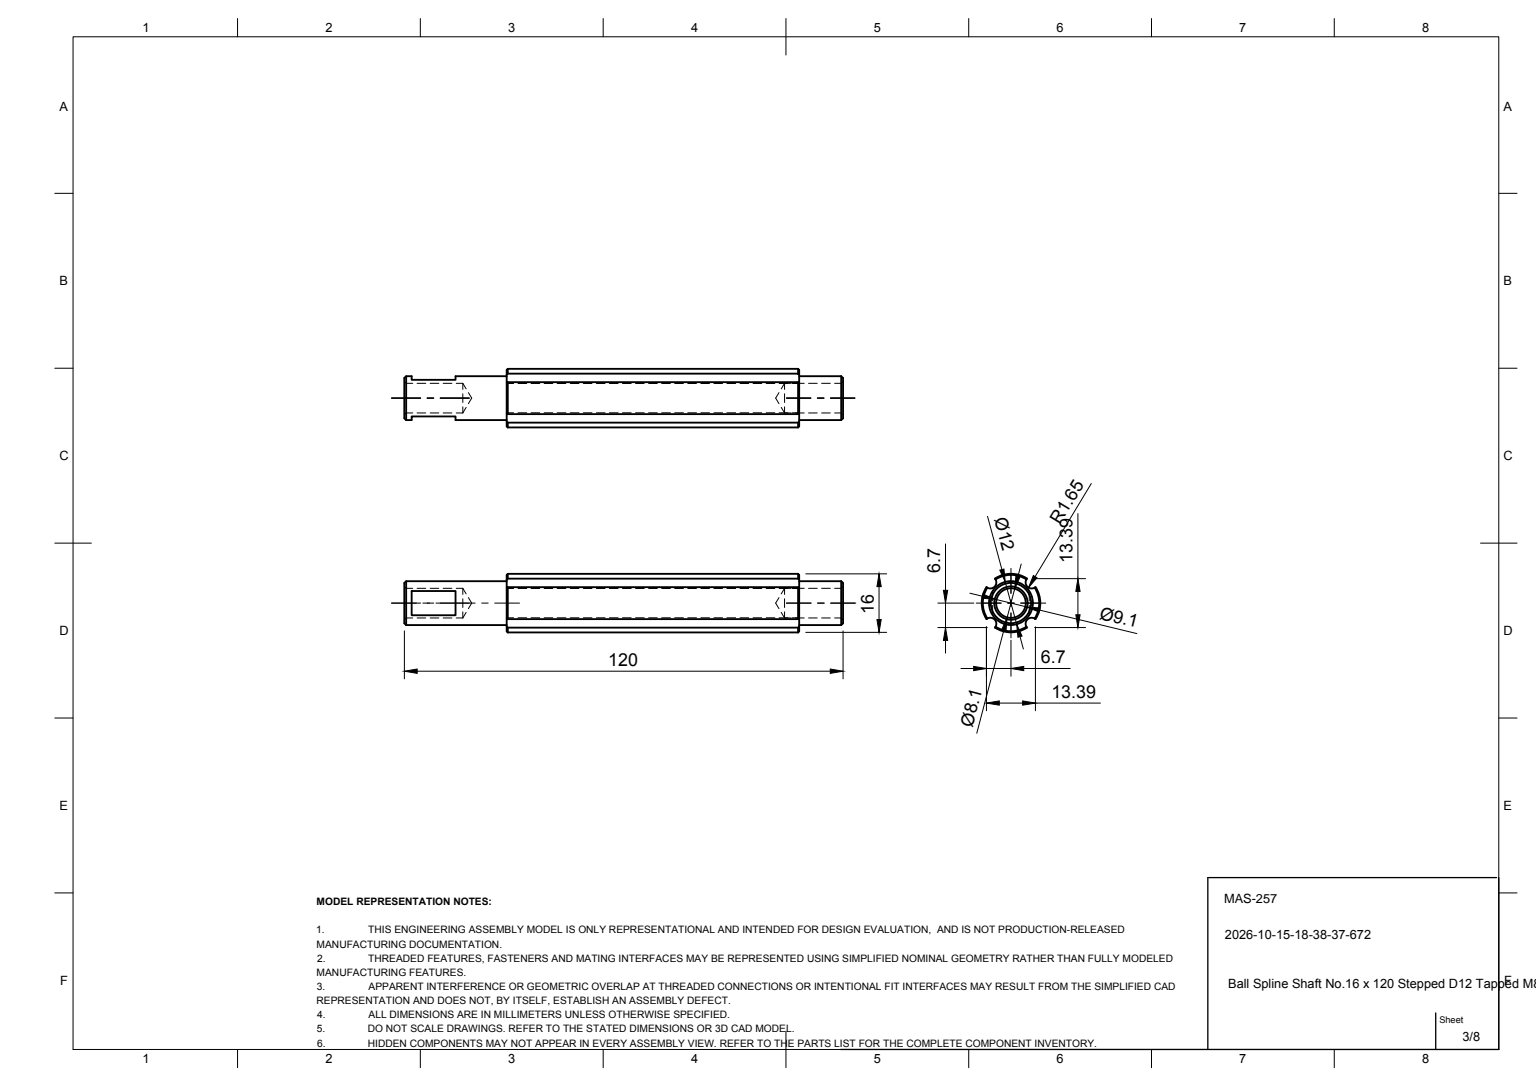
ISO-10303-21;
HEADER;
FILE_DESCRIPTION((''),'2;1');
FILE_NAME('Ball Spline Shaft No.16 x 120 Stepped D12 Tapped M8.step','2026-10-05T22:33:56+05:00',(''),(''),'','','');
FILE_SCHEMA (('AUTOMOTIVE_DESIGN { 1 0 10303 214 3 1 1 }'));
ENDSEC;
DATA;
#10=MECHANICAL_DESIGN_GEOMETRIC_PRESENTATION_REPRESENTATION('',(#429),#16942);
#415=SHAPE_REPRESENTATION_RELATIONSHIP('SRR','None',#17019,#422) ;
#422=ADVANCED_BREP_SHAPE_REPRESENTATION('',(#436),#16935) ;
#429=STYLED_ITEM('',(#17063),#436) ;
#436=MANIFOLD_SOLID_BREP(
'Ball Spline Shaft No.16 x 120 Stepped D12 Tapped M8',#8178) ;
#443=B_SPLINE_CURVE_WITH_KNOTS('',3,(#11023,#11024,#11025,#11026,#11027,
#11028),.UNSPECIFIED.,.F.,.F.,(4,2,4),(0.509460619201912,0.527252628402487,
0.551151897029291),.UNSPECIFIED.) ;
#444=B_SPLINE_CURVE_WITH_KNOTS('',3,(#11032,#11033,#11034,#11035,#11036,
#11037,#11038),.UNSPECIFIED.,.F.,.F.,(4,3,4),(-0.0238992690166207,0.,0.0177920092005774),
 .UNSPECIFIED.) ;
#445=B_SPLINE_CURVE_WITH_KNOTS('',3,(#11042,#11043,#11044,#11045,#11046,
#11047,#11048),.UNSPECIFIED.,.F.,.F.,(4,3,4),(-0.0177920090905049,0.,0.0238992686268042),
 .UNSPECIFIED.) ;
#446=B_SPLINE_CURVE_WITH_KNOTS('',3,(#11052,#11053,#11054,#11055,#11056,
#11057),.UNSPECIFIED.,.F.,.F.,(4,2,4),(0.660208716959523,0.684107985586327,
0.701899994786901),.UNSPECIFIED.) ;
#447=B_SPLINE_CURVE_WITH_KNOTS('',3,(#11062,#11063,#11064,#11065,#11066,
#11067),.UNSPECIFIED.,.F.,.F.,(4,2,4),(0.509460619201911,0.527252628402487,
0.55115189702929),.UNSPECIFIED.) ;
#448=B_SPLINE_CURVE_WITH_KNOTS('',3,(#11071,#11072,#11073,#11074,#11075,
#11076,#11077),.UNSPECIFIED.,.F.,.F.,(4,3,4),(-0.0238992690166204,0.,0.0177920092005756),
 .UNSPECIFIED.) ;
#449=B_SPLINE_CURVE_WITH_KNOTS('',3,(#11081,#11082,#11083,#11084,#11085,
#11086,#11087),.UNSPECIFIED.,.F.,.F.,(4,3,4),(-0.0177920090905051,0.,0.0238992686268041),
 .UNSPECIFIED.) ;
#450=B_SPLINE_CURVE_WITH_KNOTS('',3,(#11091,#11092,#11093,#11094,#11095,
#11096),.UNSPECIFIED.,.F.,.F.,(4,2,4),(0.660208716959522,0.684107985586326,
0.701899994786901),.UNSPECIFIED.) ;
#451=B_SPLINE_CURVE_WITH_KNOTS('',3,(#11101,#11102,#11103,#11104,#11105,
#11106,#11107),.UNSPECIFIED.,.F.,.F.,(4,3,4),(-0.0238992690166182,0.,0.0177920092005759),
 .UNSPECIFIED.) ;
#452=B_SPLINE_CURVE_WITH_KNOTS('',3,(#11111,#11112,#11113,#11114,#11115,
#11116,#11117),.UNSPECIFIED.,.F.,.F.,(4,3,4),(-0.0177920090905041,0.,0.0238992686268048),
 .UNSPECIFIED.) ;
#453=B_SPLINE_CURVE_WITH_KNOTS('',3,(#11121,#11122,#11123,#11124,#11125,
#11126),.UNSPECIFIED.,.F.,.F.,(4,2,4),(0.660208716959521,0.684107985586326,
0.701899994786899),.UNSPECIFIED.) ;
#454=B_SPLINE_CURVE_WITH_KNOTS('',3,(#11130,#11131,#11132,#11133,#11134,
#11135),.UNSPECIFIED.,.F.,.F.,(4,2,4),(0.509460619201914,0.52725262840249,
0.551151897029293),.UNSPECIFIED.) ;
#455=B_SPLINE_CURVE_WITH_KNOTS('',3,(#11140,#11141,#11142,#11143,#11144,
#11145,#11146),.UNSPECIFIED.,.F.,.F.,(4,3,4),(-0.0238992690166184,0.,0.0177920092005753),
 .UNSPECIFIED.) ;
#456=B_SPLINE_CURVE_WITH_KNOTS('',3,(#11150,#11151,#11152,#11153,#11154,
#11155,#11156),.UNSPECIFIED.,.F.,.F.,(4,3,4),(-0.0177920090905042,0.,0.0238992686268048),
 .UNSPECIFIED.) ;
#457=B_SPLINE_CURVE_WITH_KNOTS('',3,(#11160,#11161,#11162,#11163,#11164,
#11165),.UNSPECIFIED.,.F.,.F.,(4,2,4),(0.660208716959522,0.684107985586326,
0.7018999947869),.UNSPECIFIED.) ;
#458=B_SPLINE_CURVE_WITH_KNOTS('',3,(#11169,#11170,#11171,#11172,#11173,
#11174),.UNSPECIFIED.,.F.,.F.,(4,2,4),(0.509460619201915,0.527252628402489,
0.551151897029294),.UNSPECIFIED.) ;
#686=FACE_BOUND('',#1506,.T.) ;
#687=FACE_BOUND('',#1511,.T.) ;
#688=FACE_BOUND('',#1536,.T.) ;
#689=FACE_BOUND('',#1540,.T.) ;
#690=FACE_BOUND('',#1542,.T.) ;
#737=PLANE('',#8271) ;
#738=PLANE('',#8280) ;
#739=PLANE('',#8283) ;
#740=PLANE('',#8286) ;
#741=PLANE('',#8287) ;
#742=PLANE('',#8290) ;
#743=PLANE('',#8292) ;
#744=PLANE('',#8293) ;
#745=PLANE('',#8335) ;
#746=PLANE('',#8340) ;
#977=CYLINDRICAL_SURFACE('',#8268,4.05) ;
#978=CYLINDRICAL_SURFACE('',#8277,4.05) ;
#979=CYLINDRICAL_SURFACE('',#8295,1.65) ;
#980=CYLINDRICAL_SURFACE('',#8298,1.65) ;
#981=CYLINDRICAL_SURFACE('',#8301,1.65) ;
#982=CYLINDRICAL_SURFACE('',#8304,1.65) ;
#983=CYLINDRICAL_SURFACE('',#8319,8.) ;
#984=CYLINDRICAL_SURFACE('',#8321,8.) ;
#985=CYLINDRICAL_SURFACE('',#8323,8.) ;
#986=CYLINDRICAL_SURFACE('',#8325,8.) ;
#987=CYLINDRICAL_SURFACE('',#8339,6.) ;
#988=CYLINDRICAL_SURFACE('',#8342,6.) ;
#1061=FACE_OUTER_BOUND('',#1503,.T.) ;
#1062=FACE_OUTER_BOUND('',#1504,.T.) ;
#1063=FACE_OUTER_BOUND('',#1505,.T.) ;
#1064=FACE_OUTER_BOUND('',#1507,.T.) ;
#1065=FACE_OUTER_BOUND('',#1508,.T.) ;
#1066=FACE_OUTER_BOUND('',#1509,.T.) ;
#1067=FACE_OUTER_BOUND('',#1510,.T.) ;
#1068=FACE_OUTER_BOUND('',#1512,.T.) ;
#1069=FACE_OUTER_BOUND('',#1513,.T.) ;
#1070=FACE_OUTER_BOUND('',#1514,.T.) ;
#1071=FACE_OUTER_BOUND('',#1515,.T.) ;
#1072=FACE_OUTER_BOUND('',#1516,.T.) ;
#1073=FACE_OUTER_BOUND('',#1517,.T.) ;
#1074=FACE_OUTER_BOUND('',#1518,.T.) ;
#1075=FACE_OUTER_BOUND('',#1519,.T.) ;
#1076=FACE_OUTER_BOUND('',#1520,.T.) ;
#1077=FACE_OUTER_BOUND('',#1521,.T.) ;
#1078=FACE_OUTER_BOUND('',#1522,.T.) ;
#1079=FACE_OUTER_BOUND('',#1523,.T.) ;
#1080=FACE_OUTER_BOUND('',#1524,.T.) ;
#1081=FACE_OUTER_BOUND('',#1525,.T.) ;
#1082=FACE_OUTER_BOUND('',#1526,.T.) ;
#1083=FACE_OUTER_BOUND('',#1527,.T.) ;
#1084=FACE_OUTER_BOUND('',#1528,.T.) ;
#1085=FACE_OUTER_BOUND('',#1529,.T.) ;
#1086=FACE_OUTER_BOUND('',#1530,.T.) ;
#1087=FACE_OUTER_BOUND('',#1531,.T.) ;
#1088=FACE_OUTER_BOUND('',#1532,.T.) ;
#1089=FACE_OUTER_BOUND('',#1533,.T.) ;
#1090=FACE_OUTER_BOUND('',#1534,.T.) ;
#1091=FACE_OUTER_BOUND('',#1535,.T.) ;
#1092=FACE_OUTER_BOUND('',#1537,.T.) ;
#1093=FACE_OUTER_BOUND('',#1538,.T.) ;
#1094=FACE_OUTER_BOUND('',#1539,.T.) ;
#1095=FACE_OUTER_BOUND('',#1541,.T.) ;
#1096=FACE_OUTER_BOUND('',#1543,.T.) ;
#1503=EDGE_LOOP('',(#5351,#5352,#5353,#5354)) ;
#1504=EDGE_LOOP('',(#5355,#5356,#5357,#5358,#5359)) ;
#1505=EDGE_LOOP('',(#5360)) ;
#1506=EDGE_LOOP('',(#5361)) ;
#1507=EDGE_LOOP('',(#5362,#5363,#5364,#5365)) ;
#1508=EDGE_LOOP('',(#5366,#5367,#5368,#5369)) ;
#1509=EDGE_LOOP('',(#5370,#5371,#5372,#5373,#5374)) ;
#1510=EDGE_LOOP('',(#5375)) ;
#1511=EDGE_LOOP('',(#5376)) ;
#1512=EDGE_LOOP('',(#5377,#5378,#5379,#5380)) ;
#1513=EDGE_LOOP('',(#5381,#5382,#5383)) ;
#1514=EDGE_LOOP('',(#5384,#5385,#5386,#5387)) ;
#1515=EDGE_LOOP('',(#5388,#5389,#5390)) ;
#1516=EDGE_LOOP('',(#5391,#5392)) ;
#1517=EDGE_LOOP('',(#5393,#5394,#5395,#5396)) ;
#1518=EDGE_LOOP('',(#5397,#5398)) ;
#1519=EDGE_LOOP('',(#5399,#5400,#5401,#5402,#5403,#5404,#5405,#5406)) ;
#1520=EDGE_LOOP('',(#5407,#5408,#5409,#5410,#5411,#5412,#5413,#5414)) ;
#1521=EDGE_LOOP('',(#5415,#5416,#5417,#5418,#5419,#5420,#5421,#5422)) ;
#1522=EDGE_LOOP('',(#5423,#5424,#5425,#5426,#5427,#5428,#5429,#5430)) ;
#1523=EDGE_LOOP('',(#5431,#5432,#5433,#5434)) ;
#1524=EDGE_LOOP('',(#5435,#5436,#5437,#5438)) ;
#1525=EDGE_LOOP('',(#5439,#5440,#5441,#5442)) ;
#1526=EDGE_LOOP('',(#5443,#5444,#5445,#5446)) ;
#1527=EDGE_LOOP('',(#5447,#5448,#5449,#5450)) ;
#1528=EDGE_LOOP('',(#5451,#5452,#5453,#5454)) ;
#1529=EDGE_LOOP('',(#5455,#5456,#5457,#5458)) ;
#1530=EDGE_LOOP('',(#5459,#5460,#5461,#5462)) ;
#1531=EDGE_LOOP('',(#5463,#5464,#5465,#5466)) ;
#1532=EDGE_LOOP('',(#5467,#5468,#5469,#5470)) ;
#1533=EDGE_LOOP('',(#5471,#5472,#5473,#5474)) ;
#1534=EDGE_LOOP('',(#5475,#5476,#5477,#5478)) ;
#1535=EDGE_LOOP('',(#5479,#5480,#5481,#5482,#5483,#5484,#5485,#5486)) ;
#1536=EDGE_LOOP('',(#5487)) ;
#1537=EDGE_LOOP('',(#5488,#5489,#5490,#5491)) ;
#1538=EDGE_LOOP('',(#5492,#5493,#5494,#5495)) ;
#1539=EDGE_LOOP('',(#5496,#5497,#5498,#5499,#5500,#5501,#5502,#5503)) ;
#1540=EDGE_LOOP('',(#5504)) ;
#1541=EDGE_LOOP('',(#5505,#5506,#5507,#5508,#5509,#5510,#5511,#5512,#5513,
#5514,#5515,#5516)) ;
#1542=EDGE_LOOP('',(#5517,#5518,#5519,#5520)) ;
#1543=EDGE_LOOP('',(#5521,#5522,#5523,#5524)) ;
#1996=LINE('',#10958,#2558) ;
#1997=LINE('',#10962,#2559) ;
#1998=LINE('',#10971,#2560) ;
#1999=LINE('',#10976,#2561) ;
#2000=LINE('',#10980,#2562) ;
#2001=LINE('',#10989,#2563) ;
#2002=LINE('',#10995,#2564) ;
#2003=LINE('',#10999,#2565) ;
#2004=LINE('',#11001,#2566) ;
#2005=LINE('',#11002,#2567) ;
#2006=LINE('',#11011,#2568) ;
#2007=LINE('',#11014,#2569) ;
#2008=LINE('',#11016,#2570) ;
#2009=LINE('',#11017,#2571) ;
#2010=LINE('',#11040,#2572) ;
#2011=LINE('',#11058,#2573) ;
#2012=LINE('',#11079,#2574) ;
#2013=LINE('',#11097,#2575) ;
#2014=LINE('',#11109,#2576) ;
#2015=LINE('',#11128,#2577) ;
#2016=LINE('',#11148,#2578) ;
#2017=LINE('',#11167,#2579) ;
#2018=LINE('',#11210,#2580) ;
#2019=LINE('',#11212,#2581) ;
#2020=LINE('',#11219,#2582) ;
#2021=LINE('',#11220,#2583) ;
#2022=LINE('',#11222,#2584) ;
#2558=VECTOR('',#8980,4.3) ;
#2559=VECTOR('',#8985,4.05) ;
#2560=VECTOR('',#8996,2.025) ;
#2561=VECTOR('',#9001,4.3) ;
#2562=VECTOR('',#9006,4.05) ;
#2563=VECTOR('',#9017,4.05) ;
#2564=VECTOR('',#9022,10.) ;
#2565=VECTOR('',#9027,10.) ;
#2566=VECTOR('',#9028,10.) ;
#2567=VECTOR('',#9029,10.) ;
#2568=VECTOR('',#9040,10.) ;
#2569=VECTOR('',#9043,10.) ;
#2570=VECTOR('',#9044,10.) ;
#2571=VECTOR('',#9045,10.) ;
#2572=VECTOR('',#9054,10.) ;
#2573=VECTOR('',#9057,10.) ;
#2574=VECTOR('',#9062,10.) ;
#2575=VECTOR('',#9065,10.) ;
#2576=VECTOR('',#9068,10.) ;
#2577=VECTOR('',#9071,10.) ;
#2578=VECTOR('',#9076,10.) ;
#2579=VECTOR('',#9079,10.) ;
#2580=VECTOR('',#9146,5.75) ;
#2581=VECTOR('',#9149,6.) ;
#2582=VECTOR('',#9158,6.) ;
#2583=VECTOR('',#9159,6.) ;
#2584=VECTOR('',#9162,5.75) ;
#3120=CIRCLE('',#8266,4.55) ;
#3121=CIRCLE('',#8267,4.05) ;
#3122=CIRCLE('',#8269,4.05) ;
#3123=CIRCLE('',#8270,4.05) ;
#3124=CIRCLE('',#8272,5.5) ;
#3125=CIRCLE('',#8275,4.55) ;
#3126=CIRCLE('',#8276,4.05) ;
#3127=CIRCLE('',#8278,4.05) ;
#3128=CIRCLE('',#8279,4.05) ;
#3129=CIRCLE('',#8281,5.5) ;
#3130=CIRCLE('',#8284,6.) ;
#3131=CIRCLE('',#8285,6.) ;
#3132=CIRCLE('',#8288,6.) ;
#3133=CIRCLE('',#8289,6.) ;
#3134=CIRCLE('',#8291,6.) ;
#3135=CIRCLE('',#8294,6.) ;
#3136=CIRCLE('',#8296,1.65) ;
#3137=CIRCLE('',#8297,1.65) ;
#3138=CIRCLE('',#8299,1.65) ;
#3139=CIRCLE('',#8300,1.65) ;
#3140=CIRCLE('',#8302,1.65) ;
#3141=CIRCLE('',#8303,1.65) ;
#3142=CIRCLE('',#8305,1.65) ;
#3143=CIRCLE('',#8306,1.65) ;
#3144=CIRCLE('',#8308,8.) ;
#3145=CIRCLE('',#8309,7.7) ;
#3146=CIRCLE('',#8311,8.) ;
#3147=CIRCLE('',#8312,7.7) ;
#3148=CIRCLE('',#8314,7.7) ;
#3149=CIRCLE('',#8315,8.) ;
#3150=CIRCLE('',#8317,8.) ;
#3151=CIRCLE('',#8318,7.7) ;
#3152=CIRCLE('',#8320,8.) ;
#3153=CIRCLE('',#8322,8.) ;
#3154=CIRCLE('',#8324,8.) ;
#3155=CIRCLE('',#8326,8.) ;
#3156=CIRCLE('',#8328,7.7) ;
#3157=CIRCLE('',#8330,7.7) ;
#3158=CIRCLE('',#8332,7.7) ;
#3159=CIRCLE('',#8334,7.7) ;
#3160=CIRCLE('',#8336,6.) ;
#3161=CIRCLE('',#8338,6.) ;
#3162=CIRCLE('',#8341,6.) ;
#3163=CIRCLE('',#8343,6.) ;
#3398=VERTEX_POINT('',#10955) ;
#3399=VERTEX_POINT('',#10957) ;
#3400=VERTEX_POINT('',#10961) ;
#3401=VERTEX_POINT('',#10963) ;
#3402=VERTEX_POINT('',#10967) ;
#3403=VERTEX_POINT('',#10970) ;
#3404=VERTEX_POINT('',#10973) ;
#3405=VERTEX_POINT('',#10975) ;
#3406=VERTEX_POINT('',#10979) ;
#3407=VERTEX_POINT('',#10981) ;
#3408=VERTEX_POINT('',#10985) ;
#3409=VERTEX_POINT('',#10988) ;
#3410=VERTEX_POINT('',#10991) ;
#3411=VERTEX_POINT('',#10992) ;
#3412=VERTEX_POINT('',#10994) ;
#3413=VERTEX_POINT('',#10998) ;
#3414=VERTEX_POINT('',#11000) ;
#3415=VERTEX_POINT('',#11004) ;
#3416=VERTEX_POINT('',#11008) ;
#3417=VERTEX_POINT('',#11009) ;
#3418=VERTEX_POINT('',#11013) ;
#3419=VERTEX_POINT('',#11015) ;
#3420=VERTEX_POINT('',#11021) ;
#3421=VERTEX_POINT('',#11022) ;
#3422=VERTEX_POINT('',#11029) ;
#3423=VERTEX_POINT('',#11031) ;
#3424=VERTEX_POINT('',#11039) ;
#3425=VERTEX_POINT('',#11041) ;
#3426=VERTEX_POINT('',#11049) ;
#3427=VERTEX_POINT('',#11051) ;
#3428=VERTEX_POINT('',#11060) ;
#3429=VERTEX_POINT('',#11061) ;
#3430=VERTEX_POINT('',#11068) ;
#3431=VERTEX_POINT('',#11070) ;
#3432=VERTEX_POINT('',#11078) ;
#3433=VERTEX_POINT('',#11080) ;
#3434=VERTEX_POINT('',#11088) ;
#3435=VERTEX_POINT('',#11090) ;
#3436=VERTEX_POINT('',#11099) ;
#3437=VERTEX_POINT('',#11100) ;
#3438=VERTEX_POINT('',#11108) ;
#3439=VERTEX_POINT('',#11110) ;
#3440=VERTEX_POINT('',#11118) ;
#3441=VERTEX_POINT('',#11120) ;
#3442=VERTEX_POINT('',#11127) ;
#3443=VERTEX_POINT('',#11129) ;
#3444=VERTEX_POINT('',#11138) ;
#3445=VERTEX_POINT('',#11139) ;
#3446=VERTEX_POINT('',#11147) ;
#3447=VERTEX_POINT('',#11149) ;
#3448=VERTEX_POINT('',#11157) ;
#3449=VERTEX_POINT('',#11159) ;
#3450=VERTEX_POINT('',#11166) ;
#3451=VERTEX_POINT('',#11168) ;
#3452=VERTEX_POINT('',#11205) ;
#3453=VERTEX_POINT('',#11208) ;
#3454=VERTEX_POINT('',#11214) ;
#3455=VERTEX_POINT('',#11217) ;
#4173=EDGE_CURVE('',#3398,#3398,#3120,.T.) ;
#4174=EDGE_CURVE('',#3398,#3399,#1996,.T.) ;
#4175=EDGE_CURVE('',#3399,#3399,#3121,.T.) ;
#4176=EDGE_CURVE('',#3399,#3400,#1997,.T.) ;
#4177=EDGE_CURVE('',#3400,#3401,#3122,.T.) ;
#4178=EDGE_CURVE('',#3401,#3400,#3123,.T.) ;
#4179=EDGE_CURVE('',#3402,#3402,#3124,.T.) ;
#4180=EDGE_CURVE('',#3403,#3401,#1998,.T.) ;
#4181=EDGE_CURVE('',#3404,#3404,#3125,.T.) ;
#4182=EDGE_CURVE('',#3404,#3405,#1999,.T.) ;
#4183=EDGE_CURVE('',#3405,#3405,#3126,.T.) ;
#4184=EDGE_CURVE('',#3405,#3406,#2000,.T.) ;
#4185=EDGE_CURVE('',#3406,#3407,#3127,.T.) ;
#4186=EDGE_CURVE('',#3407,#3406,#3128,.T.) ;
#4187=EDGE_CURVE('',#3408,#3408,#3129,.T.) ;
#4188=EDGE_CURVE('',#3407,#3409,#2001,.T.) ;
#4189=EDGE_CURVE('',#3410,#3411,#3130,.T.) ;
#4190=EDGE_CURVE('',#3412,#3410,#2002,.T.) ;
#4191=EDGE_CURVE('',#3411,#3412,#3131,.T.) ;
#4192=EDGE_CURVE('',#3413,#3410,#2003,.T.) ;
#4193=EDGE_CURVE('',#3413,#3414,#2004,.T.) ;
#4194=EDGE_CURVE('',#3412,#3414,#2005,.T.) ;
#4195=EDGE_CURVE('',#3414,#3415,#3132,.T.) ;
#4196=EDGE_CURVE('',#3415,#3413,#3133,.T.) ;
#4197=EDGE_CURVE('',#3416,#3417,#3134,.T.) ;
#4198=EDGE_CURVE('',#3416,#3417,#2006,.T.) ;
#4199=EDGE_CURVE('',#3418,#3416,#2007,.T.) ;
#4200=EDGE_CURVE('',#3418,#3419,#2008,.T.) ;
#4201=EDGE_CURVE('',#3417,#3419,#2009,.T.) ;
#4202=EDGE_CURVE('',#3419,#3418,#3135,.T.) ;
#4203=EDGE_CURVE('',#3420,#3421,#443,.T.) ;
#4204=EDGE_CURVE('',#3422,#3420,#3136,.T.) ;
#4205=EDGE_CURVE('',#3423,#3422,#444,.T.) ;
#4206=EDGE_CURVE('',#3424,#3423,#2010,.T.) ;
#4207=EDGE_CURVE('',#3425,#3424,#445,.T.) ;
#4208=EDGE_CURVE('',#3426,#3425,#3137,.T.) ;
#4209=EDGE_CURVE('',#3427,#3426,#446,.T.) ;
#4210=EDGE_CURVE('',#3421,#3427,#2011,.T.) ;
#4211=EDGE_CURVE('',#3428,#3429,#447,.T.) ;
#4212=EDGE_CURVE('',#3430,#3428,#3138,.T.) ;
#4213=EDGE_CURVE('',#3431,#3430,#448,.T.) ;
#4214=EDGE_CURVE('',#3432,#3431,#2012,.T.) ;
#4215=EDGE_CURVE('',#3433,#3432,#449,.T.) ;
#4216=EDGE_CURVE('',#3434,#3433,#3139,.T.) ;
#4217=EDGE_CURVE('',#3435,#3434,#450,.T.) ;
#4218=EDGE_CURVE('',#3429,#3435,#2013,.T.) ;
#4219=EDGE_CURVE('',#3436,#3437,#451,.T.) ;
#4220=EDGE_CURVE('',#3438,#3436,#2014,.T.) ;
#4221=EDGE_CURVE('',#3439,#3438,#452,.T.) ;
#4222=EDGE_CURVE('',#3440,#3439,#3140,.T.) ;
#4223=EDGE_CURVE('',#3441,#3440,#453,.T.) ;
#4224=EDGE_CURVE('',#3442,#3441,#2015,.T.) ;
#4225=EDGE_CURVE('',#3443,#3442,#454,.T.) ;
#4226=EDGE_CURVE('',#3437,#3443,#3141,.T.) ;
#4227=EDGE_CURVE('',#3444,#3445,#455,.T.) ;
#4228=EDGE_CURVE('',#3446,#3444,#2016,.T.) ;
#4229=EDGE_CURVE('',#3447,#3446,#456,.T.) ;
#4230=EDGE_CURVE('',#3448,#3447,#3142,.T.) ;
#4231=EDGE_CURVE('',#3449,#3448,#457,.T.) ;
#4232=EDGE_CURVE('',#3450,#3449,#2017,.T.) ;
#4233=EDGE_CURVE('',#3451,#3450,#458,.T.) ;
#4234=EDGE_CURVE('',#3445,#3451,#3143,.T.) ;
#4235=EDGE_CURVE('',#3442,#3444,#3144,.T.) ;
#4236=EDGE_CURVE('',#3443,#3445,#3145,.T.) ;
#4237=EDGE_CURVE('',#3429,#3436,#3146,.T.) ;
#4238=EDGE_CURVE('',#3428,#3437,#3147,.T.) ;
#4239=EDGE_CURVE('',#3451,#3422,#3148,.T.) ;
#4240=EDGE_CURVE('',#3450,#3423,#3149,.T.) ;
#4241=EDGE_CURVE('',#3421,#3431,#3150,.T.) ;
#4242=EDGE_CURVE('',#3420,#3430,#3151,.T.) ;
#4243=EDGE_CURVE('',#3441,#3446,#3152,.T.) ;
#4244=EDGE_CURVE('',#3435,#3438,#3153,.T.) ;
#4245=EDGE_CURVE('',#3449,#3424,#3154,.T.) ;
#4246=EDGE_CURVE('',#3427,#3432,#3155,.T.) ;
#4247=EDGE_CURVE('',#3440,#3447,#3156,.T.) ;
#4248=EDGE_CURVE('',#3434,#3439,#3157,.T.) ;
#4249=EDGE_CURVE('',#3448,#3425,#3158,.T.) ;
#4250=EDGE_CURVE('',#3426,#3433,#3159,.T.) ;
#4251=EDGE_CURVE('',#3452,#3452,#3160,.T.) ;
#4252=EDGE_CURVE('',#3453,#3453,#3161,.T.) ;
#4253=EDGE_CURVE('',#3453,#3408,#2018,.T.) ;
#4254=EDGE_CURVE('',#3452,#3453,#2019,.T.) ;
#4255=EDGE_CURVE('',#3454,#3454,#3162,.T.) ;
#4256=EDGE_CURVE('',#3455,#3455,#3163,.T.) ;
#4257=EDGE_CURVE('',#3455,#3411,#2020,.T.) ;
#4258=EDGE_CURVE('',#3415,#3454,#2021,.T.) ;
#4259=EDGE_CURVE('',#3402,#3455,#2022,.T.) ;
#5351=ORIENTED_EDGE('',*,*,#4173,.T.) ;
#5352=ORIENTED_EDGE('',*,*,#4174,.T.) ;
#5353=ORIENTED_EDGE('',*,*,#4175,.T.) ;
#5354=ORIENTED_EDGE('',*,*,#4174,.F.) ;
#5355=ORIENTED_EDGE('',*,*,#4175,.F.) ;
#5356=ORIENTED_EDGE('',*,*,#4176,.T.) ;
#5357=ORIENTED_EDGE('',*,*,#4177,.T.) ;
#5358=ORIENTED_EDGE('',*,*,#4178,.T.) ;
#5359=ORIENTED_EDGE('',*,*,#4176,.F.) ;
#5360=ORIENTED_EDGE('',*,*,#4179,.T.) ;
#5361=ORIENTED_EDGE('',*,*,#4173,.F.) ;
#5362=ORIENTED_EDGE('',*,*,#4180,.T.) ;
#5363=ORIENTED_EDGE('',*,*,#4177,.F.) ;
#5364=ORIENTED_EDGE('',*,*,#4178,.F.) ;
#5365=ORIENTED_EDGE('',*,*,#4180,.F.) ;
#5366=ORIENTED_EDGE('',*,*,#4181,.T.) ;
#5367=ORIENTED_EDGE('',*,*,#4182,.T.) ;
#5368=ORIENTED_EDGE('',*,*,#4183,.T.) ;
#5369=ORIENTED_EDGE('',*,*,#4182,.F.) ;
#5370=ORIENTED_EDGE('',*,*,#4183,.F.) ;
#5371=ORIENTED_EDGE('',*,*,#4184,.T.) ;
#5372=ORIENTED_EDGE('',*,*,#4185,.T.) ;
#5373=ORIENTED_EDGE('',*,*,#4186,.T.) ;
#5374=ORIENTED_EDGE('',*,*,#4184,.F.) ;
#5375=ORIENTED_EDGE('',*,*,#4187,.F.) ;
#5376=ORIENTED_EDGE('',*,*,#4181,.F.) ;
#5377=ORIENTED_EDGE('',*,*,#4186,.F.) ;
#5378=ORIENTED_EDGE('',*,*,#4188,.T.) ;
#5379=ORIENTED_EDGE('',*,*,#4188,.F.) ;
#5380=ORIENTED_EDGE('',*,*,#4185,.F.) ;
#5381=ORIENTED_EDGE('',*,*,#4189,.F.) ;
#5382=ORIENTED_EDGE('',*,*,#4190,.F.) ;
#5383=ORIENTED_EDGE('',*,*,#4191,.F.) ;
#5384=ORIENTED_EDGE('',*,*,#4192,.F.) ;
#5385=ORIENTED_EDGE('',*,*,#4193,.T.) ;
#5386=ORIENTED_EDGE('',*,*,#4194,.F.) ;
#5387=ORIENTED_EDGE('',*,*,#4190,.T.) ;
#5388=ORIENTED_EDGE('',*,*,#4195,.F.) ;
#5389=ORIENTED_EDGE('',*,*,#4193,.F.) ;
#5390=ORIENTED_EDGE('',*,*,#4196,.F.) ;
#5391=ORIENTED_EDGE('',*,*,#4197,.F.) ;
#5392=ORIENTED_EDGE('',*,*,#4198,.T.) ;
#5393=ORIENTED_EDGE('',*,*,#4199,.F.) ;
#5394=ORIENTED_EDGE('',*,*,#4200,.T.) ;
#5395=ORIENTED_EDGE('',*,*,#4201,.F.) ;
#5396=ORIENTED_EDGE('',*,*,#4198,.F.) ;
#5397=ORIENTED_EDGE('',*,*,#4202,.F.) ;
#5398=ORIENTED_EDGE('',*,*,#4200,.F.) ;
#5399=ORIENTED_EDGE('',*,*,#4203,.F.) ;
#5400=ORIENTED_EDGE('',*,*,#4204,.F.) ;
#5401=ORIENTED_EDGE('',*,*,#4205,.F.) ;
#5402=ORIENTED_EDGE('',*,*,#4206,.F.) ;
#5403=ORIENTED_EDGE('',*,*,#4207,.F.) ;
#5404=ORIENTED_EDGE('',*,*,#4208,.F.) ;
#5405=ORIENTED_EDGE('',*,*,#4209,.F.) ;
#5406=ORIENTED_EDGE('',*,*,#4210,.F.) ;
#5407=ORIENTED_EDGE('',*,*,#4211,.F.) ;
#5408=ORIENTED_EDGE('',*,*,#4212,.F.) ;
#5409=ORIENTED_EDGE('',*,*,#4213,.F.) ;
#5410=ORIENTED_EDGE('',*,*,#4214,.F.) ;
#5411=ORIENTED_EDGE('',*,*,#4215,.F.) ;
#5412=ORIENTED_EDGE('',*,*,#4216,.F.) ;
#5413=ORIENTED_EDGE('',*,*,#4217,.F.) ;
#5414=ORIENTED_EDGE('',*,*,#4218,.F.) ;
#5415=ORIENTED_EDGE('',*,*,#4219,.F.) ;
#5416=ORIENTED_EDGE('',*,*,#4220,.F.) ;
#5417=ORIENTED_EDGE('',*,*,#4221,.F.) ;
#5418=ORIENTED_EDGE('',*,*,#4222,.F.) ;
#5419=ORIENTED_EDGE('',*,*,#4223,.F.) ;
#5420=ORIENTED_EDGE('',*,*,#4224,.F.) ;
#5421=ORIENTED_EDGE('',*,*,#4225,.F.) ;
#5422=ORIENTED_EDGE('',*,*,#4226,.F.) ;
#5423=ORIENTED_EDGE('',*,*,#4227,.F.) ;
#5424=ORIENTED_EDGE('',*,*,#4228,.F.) ;
#5425=ORIENTED_EDGE('',*,*,#4229,.F.) ;
#5426=ORIENTED_EDGE('',*,*,#4230,.F.) ;
#5427=ORIENTED_EDGE('',*,*,#4231,.F.) ;
#5428=ORIENTED_EDGE('',*,*,#4232,.F.) ;
#5429=ORIENTED_EDGE('',*,*,#4233,.F.) ;
#5430=ORIENTED_EDGE('',*,*,#4234,.F.) ;
#5431=ORIENTED_EDGE('',*,*,#4225,.T.) ;
#5432=ORIENTED_EDGE('',*,*,#4235,.T.) ;
#5433=ORIENTED_EDGE('',*,*,#4227,.T.) ;
#5434=ORIENTED_EDGE('',*,*,#4236,.F.) ;
#5435=ORIENTED_EDGE('',*,*,#4211,.T.) ;
#5436=ORIENTED_EDGE('',*,*,#4237,.T.) ;
#5437=ORIENTED_EDGE('',*,*,#4219,.T.) ;
#5438=ORIENTED_EDGE('',*,*,#4238,.F.) ;
#5439=ORIENTED_EDGE('',*,*,#4205,.T.) ;
#5440=ORIENTED_EDGE('',*,*,#4239,.F.) ;
#5441=ORIENTED_EDGE('',*,*,#4233,.T.) ;
#5442=ORIENTED_EDGE('',*,*,#4240,.T.) ;
#5443=ORIENTED_EDGE('',*,*,#4203,.T.) ;
#5444=ORIENTED_EDGE('',*,*,#4241,.T.) ;
#5445=ORIENTED_EDGE('',*,*,#4213,.T.) ;
#5446=ORIENTED_EDGE('',*,*,#4242,.F.) ;
#5447=ORIENTED_EDGE('',*,*,#4224,.T.) ;
#5448=ORIENTED_EDGE('',*,*,#4243,.T.) ;
#5449=ORIENTED_EDGE('',*,*,#4228,.T.) ;
#5450=ORIENTED_EDGE('',*,*,#4235,.F.) ;
#5451=ORIENTED_EDGE('',*,*,#4218,.T.) ;
#5452=ORIENTED_EDGE('',*,*,#4244,.T.) ;
#5453=ORIENTED_EDGE('',*,*,#4220,.T.) ;
#5454=ORIENTED_EDGE('',*,*,#4237,.F.) ;
#5455=ORIENTED_EDGE('',*,*,#4206,.T.) ;
#5456=ORIENTED_EDGE('',*,*,#4240,.F.) ;
#5457=ORIENTED_EDGE('',*,*,#4232,.T.) ;
#5458=ORIENTED_EDGE('',*,*,#4245,.T.) ;
#5459=ORIENTED_EDGE('',*,*,#4210,.T.) ;
#5460=ORIENTED_EDGE('',*,*,#4246,.T.) ;
#5461=ORIENTED_EDGE('',*,*,#4214,.T.) ;
#5462=ORIENTED_EDGE('',*,*,#4241,.F.) ;
#5463=ORIENTED_EDGE('',*,*,#4223,.T.) ;
#5464=ORIENTED_EDGE('',*,*,#4247,.T.) ;
#5465=ORIENTED_EDGE('',*,*,#4229,.T.) ;
#5466=ORIENTED_EDGE('',*,*,#4243,.F.) ;
#5467=ORIENTED_EDGE('',*,*,#4217,.T.) ;
#5468=ORIENTED_EDGE('',*,*,#4248,.T.) ;
#5469=ORIENTED_EDGE('',*,*,#4221,.T.) ;
#5470=ORIENTED_EDGE('',*,*,#4244,.F.) ;
#5471=ORIENTED_EDGE('',*,*,#4207,.T.) ;
#5472=ORIENTED_EDGE('',*,*,#4245,.F.) ;
#5473=ORIENTED_EDGE('',*,*,#4231,.T.) ;
#5474=ORIENTED_EDGE('',*,*,#4249,.T.) ;
#5475=ORIENTED_EDGE('',*,*,#4209,.T.) ;
#5476=ORIENTED_EDGE('',*,*,#4250,.T.) ;
#5477=ORIENTED_EDGE('',*,*,#4215,.T.) ;
#5478=ORIENTED_EDGE('',*,*,#4246,.F.) ;
#5479=ORIENTED_EDGE('',*,*,#4208,.T.) ;
#5480=ORIENTED_EDGE('',*,*,#4249,.F.) ;
#5481=ORIENTED_EDGE('',*,*,#4230,.T.) ;
#5482=ORIENTED_EDGE('',*,*,#4247,.F.) ;
#5483=ORIENTED_EDGE('',*,*,#4222,.T.) ;
#5484=ORIENTED_EDGE('',*,*,#4248,.F.) ;
#5485=ORIENTED_EDGE('',*,*,#4216,.T.) ;
#5486=ORIENTED_EDGE('',*,*,#4250,.F.) ;
#5487=ORIENTED_EDGE('',*,*,#4251,.T.) ;
#5488=ORIENTED_EDGE('',*,*,#4252,.F.) ;
#5489=ORIENTED_EDGE('',*,*,#4253,.T.) ;
#5490=ORIENTED_EDGE('',*,*,#4187,.T.) ;
#5491=ORIENTED_EDGE('',*,*,#4253,.F.) ;
#5492=ORIENTED_EDGE('',*,*,#4251,.F.) ;
#5493=ORIENTED_EDGE('',*,*,#4254,.T.) ;
#5494=ORIENTED_EDGE('',*,*,#4252,.T.) ;
#5495=ORIENTED_EDGE('',*,*,#4254,.F.) ;
#5496=ORIENTED_EDGE('',*,*,#4204,.T.) ;
#5497=ORIENTED_EDGE('',*,*,#4242,.T.) ;
#5498=ORIENTED_EDGE('',*,*,#4212,.T.) ;
#5499=ORIENTED_EDGE('',*,*,#4238,.T.) ;
#5500=ORIENTED_EDGE('',*,*,#4226,.T.) ;
#5501=ORIENTED_EDGE('',*,*,#4236,.T.) ;
#5502=ORIENTED_EDGE('',*,*,#4234,.T.) ;
#5503=ORIENTED_EDGE('',*,*,#4239,.T.) ;
#5504=ORIENTED_EDGE('',*,*,#4255,.F.) ;
#5505=ORIENTED_EDGE('',*,*,#4256,.F.) ;
#5506=ORIENTED_EDGE('',*,*,#4257,.T.) ;
#5507=ORIENTED_EDGE('',*,*,#4191,.T.) ;
#5508=ORIENTED_EDGE('',*,*,#4194,.T.) ;
#5509=ORIENTED_EDGE('',*,*,#4195,.T.) ;
#5510=ORIENTED_EDGE('',*,*,#4258,.T.) ;
#5511=ORIENTED_EDGE('',*,*,#4255,.T.) ;
#5512=ORIENTED_EDGE('',*,*,#4258,.F.) ;
#5513=ORIENTED_EDGE('',*,*,#4196,.T.) ;
#5514=ORIENTED_EDGE('',*,*,#4192,.T.) ;
#5515=ORIENTED_EDGE('',*,*,#4189,.T.) ;
#5516=ORIENTED_EDGE('',*,*,#4257,.F.) ;
#5517=ORIENTED_EDGE('',*,*,#4201,.T.) ;
#5518=ORIENTED_EDGE('',*,*,#4202,.T.) ;
#5519=ORIENTED_EDGE('',*,*,#4199,.T.) ;
#5520=ORIENTED_EDGE('',*,*,#4197,.T.) ;
#5521=ORIENTED_EDGE('',*,*,#4179,.F.) ;
#5522=ORIENTED_EDGE('',*,*,#4259,.T.) ;
#5523=ORIENTED_EDGE('',*,*,#4256,.T.) ;
#5524=ORIENTED_EDGE('',*,*,#4259,.F.) ;
#7707=CONICAL_SURFACE('',#8265,4.3,0.785398163397439) ;
#7708=CONICAL_SURFACE('',#8273,2.025,1.02974425867665) ;
#7709=CONICAL_SURFACE('',#8274,4.3,0.785398163397447) ;
#7710=CONICAL_SURFACE('',#8282,4.05,1.02974425867666) ;
#7711=CONICAL_SURFACE('',#8307,7.85,0.785398163397456) ;
#7712=CONICAL_SURFACE('',#8310,7.85,0.785398163397456) ;
#7713=CONICAL_SURFACE('',#8313,7.85,0.785398163397456) ;
#7714=CONICAL_SURFACE('',#8316,7.85,0.785398163397456) ;
#7715=CONICAL_SURFACE('',#8327,7.85,0.785398163397445) ;
#7716=CONICAL_SURFACE('',#8329,7.85,0.785398163397445) ;
#7717=CONICAL_SURFACE('',#8331,7.85,0.785398163397445) ;
#7718=CONICAL_SURFACE('',#8333,7.85,0.785398163397445) ;
#7719=CONICAL_SURFACE('',#8337,5.75,0.785398163397447) ;
#7720=CONICAL_SURFACE('',#8344,5.75,0.785398163397439) ;
#7736=ADVANCED_FACE('',(#1061),#7707,.F.) ;
#7737=ADVANCED_FACE('',(#1062),#977,.F.) ;
#7738=ADVANCED_FACE('',(#1063,#686),#737,.T.) ;
#7739=ADVANCED_FACE('',(#1064),#7708,.F.) ;
#7740=ADVANCED_FACE('',(#1065),#7709,.F.) ;
#7741=ADVANCED_FACE('',(#1066),#978,.F.) ;
#7742=ADVANCED_FACE('',(#1067,#687),#738,.T.) ;
#7743=ADVANCED_FACE('',(#1068),#7710,.F.) ;
#7744=ADVANCED_FACE('',(#1069),#739,.F.) ;
#7745=ADVANCED_FACE('',(#1070),#740,.F.) ;
#7746=ADVANCED_FACE('',(#1071),#741,.T.) ;
#7747=ADVANCED_FACE('',(#1072),#742,.T.) ;
#7748=ADVANCED_FACE('',(#1073),#743,.F.) ;
#7749=ADVANCED_FACE('',(#1074),#744,.F.) ;
#7750=ADVANCED_FACE('',(#1075),#979,.F.) ;
#7751=ADVANCED_FACE('',(#1076),#980,.F.) ;
#7752=ADVANCED_FACE('',(#1077),#981,.F.) ;
#7753=ADVANCED_FACE('',(#1078),#982,.F.) ;
#7754=ADVANCED_FACE('',(#1079),#7711,.T.) ;
#7755=ADVANCED_FACE('',(#1080),#7712,.T.) ;
#7756=ADVANCED_FACE('',(#1081),#7713,.T.) ;
#7757=ADVANCED_FACE('',(#1082),#7714,.T.) ;
#7758=ADVANCED_FACE('',(#1083),#983,.T.) ;
#7759=ADVANCED_FACE('',(#1084),#984,.T.) ;
#7760=ADVANCED_FACE('',(#1085),#985,.T.) ;
#7761=ADVANCED_FACE('',(#1086),#986,.T.) ;
#7762=ADVANCED_FACE('',(#1087),#7715,.T.) ;
#7763=ADVANCED_FACE('',(#1088),#7716,.T.) ;
#7764=ADVANCED_FACE('',(#1089),#7717,.T.) ;
#7765=ADVANCED_FACE('',(#1090),#7718,.T.) ;
#7766=ADVANCED_FACE('',(#1091,#688),#745,.T.) ;
#7767=ADVANCED_FACE('',(#1092),#7719,.T.) ;
#7768=ADVANCED_FACE('',(#1093),#987,.T.) ;
#7769=ADVANCED_FACE('',(#1094,#689),#746,.T.) ;
#7770=ADVANCED_FACE('',(#1095,#690),#988,.T.) ;
#7771=ADVANCED_FACE('',(#1096),#7720,.T.) ;
#8178=CLOSED_SHELL('',(#7736,#7737,#7738,#7739,#7740,#7741,#7742,#7743,
#7744,#7745,#7746,#7747,#7748,#7749,#7750,#7751,#7752,#7753,#7754,#7755,
#7756,#7757,#7758,#7759,#7760,#7761,#7762,#7763,#7764,#7765,#7766,#7767,
#7768,#7769,#7770,#7771)) ;
#8264=AXIS2_PLACEMENT_3D('',#10953,#8974,#8975) ;
#8265=AXIS2_PLACEMENT_3D('',#10954,#8976,#8977) ;
#8266=AXIS2_PLACEMENT_3D('',#10956,#8978,#8979) ;
#8267=AXIS2_PLACEMENT_3D('',#10959,#8981,#8982) ;
#8268=AXIS2_PLACEMENT_3D('',#10960,#8983,#8984) ;
#8269=AXIS2_PLACEMENT_3D('',#10964,#8986,#8987) ;
#8270=AXIS2_PLACEMENT_3D('',#10965,#8988,#8989) ;
#8271=AXIS2_PLACEMENT_3D('',#10966,#8990,#8991) ;
#8272=AXIS2_PLACEMENT_3D('',#10968,#8992,#8993) ;
#8273=AXIS2_PLACEMENT_3D('',#10969,#8994,#8995) ;
#8274=AXIS2_PLACEMENT_3D('',#10972,#8997,#8998) ;
#8275=AXIS2_PLACEMENT_3D('',#10974,#8999,#9000) ;
#8276=AXIS2_PLACEMENT_3D('',#10977,#9002,#9003) ;
#8277=AXIS2_PLACEMENT_3D('',#10978,#9004,#9005) ;
#8278=AXIS2_PLACEMENT_3D('',#10982,#9007,#9008) ;
#8279=AXIS2_PLACEMENT_3D('',#10983,#9009,#9010) ;
#8280=AXIS2_PLACEMENT_3D('',#10984,#9011,#9012) ;
#8281=AXIS2_PLACEMENT_3D('',#10986,#9013,#9014) ;
#8282=AXIS2_PLACEMENT_3D('',#10987,#9015,#9016) ;
#8283=AXIS2_PLACEMENT_3D('',#10990,#9018,#9019) ;
#8284=AXIS2_PLACEMENT_3D('',#10993,#9020,#9021) ;
#8285=AXIS2_PLACEMENT_3D('',#10996,#9023,#9024) ;
#8286=AXIS2_PLACEMENT_3D('',#10997,#9025,#9026) ;
#8287=AXIS2_PLACEMENT_3D('',#11003,#9030,#9031) ;
#8288=AXIS2_PLACEMENT_3D('',#11005,#9032,#9033) ;
#8289=AXIS2_PLACEMENT_3D('',#11006,#9034,#9035) ;
#8290=AXIS2_PLACEMENT_3D('',#11007,#9036,#9037) ;
#8291=AXIS2_PLACEMENT_3D('',#11010,#9038,#9039) ;
#8292=AXIS2_PLACEMENT_3D('',#11012,#9041,#9042) ;
#8293=AXIS2_PLACEMENT_3D('',#11018,#9046,#9047) ;
#8294=AXIS2_PLACEMENT_3D('',#11019,#9048,#9049) ;
#8295=AXIS2_PLACEMENT_3D('',#11020,#9050,#9051) ;
#8296=AXIS2_PLACEMENT_3D('',#11030,#9052,#9053) ;
#8297=AXIS2_PLACEMENT_3D('',#11050,#9055,#9056) ;
#8298=AXIS2_PLACEMENT_3D('',#11059,#9058,#9059) ;
#8299=AXIS2_PLACEMENT_3D('',#11069,#9060,#9061) ;
#8300=AXIS2_PLACEMENT_3D('',#11089,#9063,#9064) ;
#8301=AXIS2_PLACEMENT_3D('',#11098,#9066,#9067) ;
#8302=AXIS2_PLACEMENT_3D('',#11119,#9069,#9070) ;
#8303=AXIS2_PLACEMENT_3D('',#11136,#9072,#9073) ;
#8304=AXIS2_PLACEMENT_3D('',#11137,#9074,#9075) ;
#8305=AXIS2_PLACEMENT_3D('',#11158,#9077,#9078) ;
#8306=AXIS2_PLACEMENT_3D('',#11175,#9080,#9081) ;
#8307=AXIS2_PLACEMENT_3D('',#11176,#9082,#9083) ;
#8308=AXIS2_PLACEMENT_3D('',#11177,#9084,#9085) ;
#8309=AXIS2_PLACEMENT_3D('',#11178,#9086,#9087) ;
#8310=AXIS2_PLACEMENT_3D('',#11179,#9088,#9089) ;
#8311=AXIS2_PLACEMENT_3D('',#11180,#9090,#9091) ;
#8312=AXIS2_PLACEMENT_3D('',#11181,#9092,#9093) ;
#8313=AXIS2_PLACEMENT_3D('',#11182,#9094,#9095) ;
#8314=AXIS2_PLACEMENT_3D('',#11183,#9096,#9097) ;
#8315=AXIS2_PLACEMENT_3D('',#11184,#9098,#9099) ;
#8316=AXIS2_PLACEMENT_3D('',#11185,#9100,#9101) ;
#8317=AXIS2_PLACEMENT_3D('',#11186,#9102,#9103) ;
#8318=AXIS2_PLACEMENT_3D('',#11187,#9104,#9105) ;
#8319=AXIS2_PLACEMENT_3D('',#11188,#9106,#9107) ;
#8320=AXIS2_PLACEMENT_3D('',#11189,#9108,#9109) ;
#8321=AXIS2_PLACEMENT_3D('',#11190,#9110,#9111) ;
#8322=AXIS2_PLACEMENT_3D('',#11191,#9112,#9113) ;
#8323=AXIS2_PLACEMENT_3D('',#11192,#9114,#9115) ;
#8324=AXIS2_PLACEMENT_3D('',#11193,#9116,#9117) ;
#8325=AXIS2_PLACEMENT_3D('',#11194,#9118,#9119) ;
#8326=AXIS2_PLACEMENT_3D('',#11195,#9120,#9121) ;
#8327=AXIS2_PLACEMENT_3D('',#11196,#9122,#9123) ;
#8328=AXIS2_PLACEMENT_3D('',#11197,#9124,#9125) ;
#8329=AXIS2_PLACEMENT_3D('',#11198,#9126,#9127) ;
#8330=AXIS2_PLACEMENT_3D('',#11199,#9128,#9129) ;
#8331=AXIS2_PLACEMENT_3D('',#11200,#9130,#9131) ;
#8332=AXIS2_PLACEMENT_3D('',#11201,#9132,#9133) ;
#8333=AXIS2_PLACEMENT_3D('',#11202,#9134,#9135) ;
#8334=AXIS2_PLACEMENT_3D('',#11203,#9136,#9137) ;
#8335=AXIS2_PLACEMENT_3D('',#11204,#9138,#9139) ;
#8336=AXIS2_PLACEMENT_3D('',#11206,#9140,#9141) ;
#8337=AXIS2_PLACEMENT_3D('',#11207,#9142,#9143) ;
#8338=AXIS2_PLACEMENT_3D('',#11209,#9144,#9145) ;
#8339=AXIS2_PLACEMENT_3D('',#11211,#9147,#9148) ;
#8340=AXIS2_PLACEMENT_3D('',#11213,#9150,#9151) ;
#8341=AXIS2_PLACEMENT_3D('',#11215,#9152,#9153) ;
#8342=AXIS2_PLACEMENT_3D('',#11216,#9154,#9155) ;
#8343=AXIS2_PLACEMENT_3D('',#11218,#9156,#9157) ;
#8344=AXIS2_PLACEMENT_3D('',#11221,#9160,#9161) ;
#8974=DIRECTION('axis',(0.,0.,1.)) ;
#8975=DIRECTION('refdir',(1.,0.,0.)) ;
#8976=DIRECTION('center_axis',(1.,0.,0.)) ;
#8977=DIRECTION('ref_axis',(0.,0.,-1.)) ;
#8978=DIRECTION('center_axis',(1.,0.,0.)) ;
#8979=DIRECTION('ref_axis',(0.,0.,-1.)) ;
#8980=DIRECTION('',(-0.707106781186554,8.65956056235486E-17,-0.707106781186541)) ;
#8981=DIRECTION('center_axis',(-1.,0.,0.)) ;
#8982=DIRECTION('ref_axis',(0.,0.,-1.)) ;
#8983=DIRECTION('center_axis',(-1.,0.,0.)) ;
#8984=DIRECTION('ref_axis',(0.,0.,-1.)) ;
#8985=DIRECTION('',(-1.,0.,0.)) ;
#8986=DIRECTION('center_axis',(-1.,0.,0.)) ;
#8987=DIRECTION('ref_axis',(0.,0.,-1.)) ;
#8988=DIRECTION('center_axis',(-1.,0.,0.)) ;
#8989=DIRECTION('ref_axis',(0.,0.,-1.)) ;
#8990=DIRECTION('center_axis',(1.,0.,0.)) ;
#8991=DIRECTION('ref_axis',(0.,0.,-1.)) ;
#8992=DIRECTION('center_axis',(1.,0.,0.)) ;
#8993=DIRECTION('ref_axis',(0.,0.,-1.)) ;
#8994=DIRECTION('center_axis',(1.,0.,0.)) ;
#8995=DIRECTION('ref_axis',(0.,1.,0.)) ;
#8996=DIRECTION('',(0.515038074910055,-0.857167300702112,-1.04972719113862E-16)) ;
#8997=DIRECTION('center_axis',(-1.,0.,0.)) ;
#8998=DIRECTION('ref_axis',(0.,0.,-1.)) ;
#8999=DIRECTION('center_axis',(-1.,0.,0.)) ;
#9000=DIRECTION('ref_axis',(0.,0.,-1.)) ;
#9001=DIRECTION('',(0.707106781186549,-8.65956056235492E-17,-0.707106781186546)) ;
#9002=DIRECTION('center_axis',(1.,0.,0.)) ;
#9003=DIRECTION('ref_axis',(0.,0.,-1.)) ;
#9004=DIRECTION('center_axis',(1.,0.,0.)) ;
#9005=DIRECTION('ref_axis',(0.,0.,-1.)) ;
#9006=DIRECTION('',(1.,0.,0.)) ;
#9007=DIRECTION('center_axis',(1.,0.,0.)) ;
#9008=DIRECTION('ref_axis',(0.,0.,-1.)) ;
#9009=DIRECTION('center_axis',(1.,0.,0.)) ;
#9010=DIRECTION('ref_axis',(0.,0.,-1.)) ;
#9011=DIRECTION('center_axis',(-1.,0.,0.)) ;
#9012=DIRECTION('ref_axis',(0.,0.,1.)) ;
#9013=DIRECTION('center_axis',(1.,0.,0.)) ;
#9014=DIRECTION('ref_axis',(0.,0.,-1.)) ;
#9015=DIRECTION('center_axis',(-1.,0.,0.)) ;
#9016=DIRECTION('ref_axis',(0.,1.,0.)) ;
#9017=DIRECTION('',(0.515038074910053,0.857167300702113,1.04972719113862E-16)) ;
#9018=DIRECTION('center_axis',(1.,0.,0.)) ;
#9019=DIRECTION('ref_axis',(0.,0.,-1.)) ;
#9020=DIRECTION('center_axis',(1.,0.,0.)) ;
#9021=DIRECTION('ref_axis',(0.,1.,0.)) ;
#9022=DIRECTION('',(0.,0.,1.)) ;
#9023=DIRECTION('center_axis',(1.,0.,0.)) ;
#9024=DIRECTION('ref_axis',(0.,1.,0.)) ;
#9025=DIRECTION('center_axis',(0.,1.,0.)) ;
#9026=DIRECTION('ref_axis',(0.,0.,1.)) ;
#9027=DIRECTION('',(1.,0.,0.)) ;
#9028=DIRECTION('',(0.,0.,-1.)) ;
#9029=DIRECTION('',(-1.,0.,0.)) ;
#9030=DIRECTION('center_axis',(1.,0.,0.)) ;
#9031=DIRECTION('ref_axis',(0.,0.,-1.)) ;
#9032=DIRECTION('center_axis',(-1.,0.,0.)) ;
#9033=DIRECTION('ref_axis',(0.,1.,0.)) ;
#9034=DIRECTION('center_axis',(-1.,0.,0.)) ;
#9035=DIRECTION('ref_axis',(0.,1.,0.)) ;
#9036=DIRECTION('center_axis',(1.,0.,0.)) ;
#9037=DIRECTION('ref_axis',(0.,0.,-1.)) ;
#9038=DIRECTION('center_axis',(-1.,0.,0.)) ;
#9039=DIRECTION('ref_axis',(0.,1.,0.)) ;
#9040=DIRECTION('',(0.,0.,-1.)) ;
#9041=DIRECTION('center_axis',(0.,-1.,0.)) ;
#9042=DIRECTION('ref_axis',(0.,0.,-1.)) ;
#9043=DIRECTION('',(-1.,0.,0.)) ;
#9044=DIRECTION('',(0.,0.,-1.)) ;
#9045=DIRECTION('',(1.,0.,0.)) ;
#9046=DIRECTION('center_axis',(1.,0.,0.)) ;
#9047=DIRECTION('ref_axis',(0.,0.,-1.)) ;
#9048=DIRECTION('center_axis',(1.,0.,0.)) ;
#9049=DIRECTION('ref_axis',(0.,1.,0.)) ;
#9050=DIRECTION('center_axis',(1.,0.,0.)) ;
#9051=DIRECTION('ref_axis',(0.,0.707106781186547,0.707106781186548)) ;
#9052=DIRECTION('center_axis',(-1.,0.,0.)) ;
#9053=DIRECTION('ref_axis',(0.,0.,-1.)) ;
#9054=DIRECTION('',(1.,0.,0.)) ;
#9055=DIRECTION('center_axis',(1.,0.,0.)) ;
#9056=DIRECTION('ref_axis',(0.,0.,-1.)) ;
#9057=DIRECTION('',(-1.,0.,0.)) ;
#9058=DIRECTION('center_axis',(1.,0.,0.)) ;
#9059=DIRECTION('ref_axis',(0.,-0.707106781186547,0.707106781186548)) ;
#9060=DIRECTION('center_axis',(-1.,0.,0.)) ;
#9061=DIRECTION('ref_axis',(0.,0.,-1.)) ;
#9062=DIRECTION('',(1.,0.,0.)) ;
#9063=DIRECTION('center_axis',(1.,0.,0.)) ;
#9064=DIRECTION('ref_axis',(0.,0.,-1.)) ;
#9065=DIRECTION('',(-1.,0.,0.)) ;
#9066=DIRECTION('center_axis',(1.,0.,0.)) ;
#9067=DIRECTION('ref_axis',(0.,0.,-1.)) ;
#9068=DIRECTION('',(1.,0.,0.)) ;
#9069=DIRECTION('center_axis',(1.,0.,0.)) ;
#9070=DIRECTION('ref_axis',(0.,0.,-1.)) ;
#9071=DIRECTION('',(-1.,0.,0.)) ;
#9072=DIRECTION('center_axis',(-1.,0.,0.)) ;
#9073=DIRECTION('ref_axis',(0.,0.,-1.)) ;
#9074=DIRECTION('center_axis',(1.,0.,0.)) ;
#9075=DIRECTION('ref_axis',(0.,0.,-1.)) ;
#9076=DIRECTION('',(1.,0.,0.)) ;
#9077=DIRECTION('center_axis',(1.,0.,0.)) ;
#9078=DIRECTION('ref_axis',(0.,0.,-1.)) ;
#9079=DIRECTION('',(-1.,0.,0.)) ;
#9080=DIRECTION('center_axis',(-1.,0.,0.)) ;
#9081=DIRECTION('ref_axis',(0.,0.,-1.)) ;
#9082=DIRECTION('center_axis',(-1.,0.,0.)) ;
#9083=DIRECTION('ref_axis',(0.,1.,0.)) ;
#9084=DIRECTION('center_axis',(1.,0.,0.)) ;
#9085=DIRECTION('ref_axis',(0.,0.,-1.)) ;
#9086=DIRECTION('center_axis',(1.,0.,0.)) ;
#9087=DIRECTION('ref_axis',(0.,0.,-1.)) ;
#9088=DIRECTION('center_axis',(-1.,0.,0.)) ;
#9089=DIRECTION('ref_axis',(0.,1.,0.)) ;
#9090=DIRECTION('center_axis',(1.,0.,0.)) ;
#9091=DIRECTION('ref_axis',(0.,0.,-1.)) ;
#9092=DIRECTION('center_axis',(1.,0.,0.)) ;
#9093=DIRECTION('ref_axis',(0.,0.,-1.)) ;
#9094=DIRECTION('center_axis',(-1.,0.,0.)) ;
#9095=DIRECTION('ref_axis',(0.,-1.,-1.01064309961486E-15)) ;
#9096=DIRECTION('center_axis',(1.,0.,0.)) ;
#9097=DIRECTION('ref_axis',(0.,0.,-1.)) ;
#9098=DIRECTION('center_axis',(1.,0.,0.)) ;
#9099=DIRECTION('ref_axis',(0.,0.,-1.)) ;
#9100=DIRECTION('center_axis',(-1.,0.,0.)) ;
#9101=DIRECTION('ref_axis',(0.,1.,0.)) ;
#9102=DIRECTION('center_axis',(1.,0.,0.)) ;
#9103=DIRECTION('ref_axis',(0.,0.,-1.)) ;
#9104=DIRECTION('center_axis',(1.,0.,0.)) ;
#9105=DIRECTION('ref_axis',(0.,0.,-1.)) ;
#9106=DIRECTION('center_axis',(1.,0.,0.)) ;
#9107=DIRECTION('ref_axis',(0.,1.,0.)) ;
#9108=DIRECTION('center_axis',(1.,0.,0.)) ;
#9109=DIRECTION('ref_axis',(0.,0.,-1.)) ;
#9110=DIRECTION('center_axis',(1.,0.,0.)) ;
#9111=DIRECTION('ref_axis',(0.,1.,0.)) ;
#9112=DIRECTION('center_axis',(1.,0.,0.)) ;
#9113=DIRECTION('ref_axis',(0.,0.,-1.)) ;
#9114=DIRECTION('center_axis',(1.,0.,0.)) ;
#9115=DIRECTION('ref_axis',(0.,-1.,-1.01064309961486E-15)) ;
#9116=DIRECTION('center_axis',(1.,0.,0.)) ;
#9117=DIRECTION('ref_axis',(0.,0.,-1.)) ;
#9118=DIRECTION('center_axis',(1.,0.,0.)) ;
#9119=DIRECTION('ref_axis',(0.,1.,0.)) ;
#9120=DIRECTION('center_axis',(1.,0.,0.)) ;
#9121=DIRECTION('ref_axis',(0.,0.,-1.)) ;
#9122=DIRECTION('center_axis',(1.,0.,0.)) ;
#9123=DIRECTION('ref_axis',(0.,1.,0.)) ;
#9124=DIRECTION('center_axis',(1.,0.,0.)) ;
#9125=DIRECTION('ref_axis',(0.,0.,-1.)) ;
#9126=DIRECTION('center_axis',(1.,0.,0.)) ;
#9127=DIRECTION('ref_axis',(0.,1.,0.)) ;
#9128=DIRECTION('center_axis',(1.,0.,0.)) ;
#9129=DIRECTION('ref_axis',(0.,0.,-1.)) ;
#9130=DIRECTION('center_axis',(1.,0.,0.)) ;
#9131=DIRECTION('ref_axis',(0.,-1.,-1.01064309961486E-15)) ;
#9132=DIRECTION('center_axis',(1.,0.,0.)) ;
#9133=DIRECTION('ref_axis',(0.,0.,-1.)) ;
#9134=DIRECTION('center_axis',(1.,0.,0.)) ;
#9135=DIRECTION('ref_axis',(0.,1.,0.)) ;
#9136=DIRECTION('center_axis',(1.,0.,0.)) ;
#9137=DIRECTION('ref_axis',(0.,0.,-1.)) ;
#9138=DIRECTION('center_axis',(-1.,0.,0.)) ;
#9139=DIRECTION('ref_axis',(0.,0.,1.)) ;
#9140=DIRECTION('center_axis',(1.,0.,0.)) ;
#9141=DIRECTION('ref_axis',(0.,0.,-1.)) ;
#9142=DIRECTION('center_axis',(1.,0.,0.)) ;
#9143=DIRECTION('ref_axis',(0.,1.,0.)) ;
#9144=DIRECTION('center_axis',(1.,0.,0.)) ;
#9145=DIRECTION('ref_axis',(0.,0.,-1.)) ;
#9146=DIRECTION('',(-0.707106781186549,0.707106781186546,8.65956056235492E-17)) ;
#9147=DIRECTION('center_axis',(1.,0.,0.)) ;
#9148=DIRECTION('ref_axis',(0.,1.,0.)) ;
#9149=DIRECTION('',(-1.,0.,0.)) ;
#9150=DIRECTION('center_axis',(1.,0.,0.)) ;
#9151=DIRECTION('ref_axis',(0.,0.,-1.)) ;
#9152=DIRECTION('center_axis',(1.,0.,0.)) ;
#9153=DIRECTION('ref_axis',(0.,0.,-1.)) ;
#9154=DIRECTION('center_axis',(1.,0.,0.)) ;
#9155=DIRECTION('ref_axis',(0.,1.,0.)) ;
#9156=DIRECTION('center_axis',(1.,0.,0.)) ;
#9157=DIRECTION('ref_axis',(0.,0.,-1.)) ;
#9158=DIRECTION('',(-1.,0.,0.)) ;
#9159=DIRECTION('',(-1.,0.,0.)) ;
#9160=DIRECTION('center_axis',(-1.,0.,0.)) ;
#9161=DIRECTION('ref_axis',(0.,1.,0.)) ;
#9162=DIRECTION('',(-0.707106781186554,-0.707106781186541,-8.65956056235486E-17)) ;
#10953=CARTESIAN_POINT('',(0.,0.,0.)) ;
#10954=CARTESIAN_POINT('Origin',(119.75,25.5,25.5)) ;
#10955=CARTESIAN_POINT('',(120.,25.5,30.05)) ;
#10956=CARTESIAN_POINT('Origin',(120.,25.5,25.5)) ;
#10957=CARTESIAN_POINT('',(119.5,25.5,29.55)) ;
#10958=CARTESIAN_POINT('',(119.75,25.5,29.8)) ;
#10959=CARTESIAN_POINT('Origin',(119.5,25.5,25.5)) ;
#10960=CARTESIAN_POINT('Origin',(120.,25.5,25.5)) ;
#10961=CARTESIAN_POINT('',(104.,25.5,29.55)) ;
#10962=CARTESIAN_POINT('',(120.,25.5,29.55)) ;
#10963=CARTESIAN_POINT('',(104.,21.45,25.5)) ;
#10964=CARTESIAN_POINT('Origin',(104.,25.5,25.5)) ;
#10965=CARTESIAN_POINT('Origin',(104.,25.5,25.5)) ;
#10966=CARTESIAN_POINT('Origin',(120.,25.5,25.5)) ;
#10967=CARTESIAN_POINT('',(120.,20.,25.5)) ;
#10968=CARTESIAN_POINT('Origin',(120.,25.5,25.5)) ;
#10969=CARTESIAN_POINT('Origin',(102.783257246469,25.5,25.5)) ;
#10970=CARTESIAN_POINT('',(101.566514492938,25.5,25.5)) ;
#10971=CARTESIAN_POINT('',(102.783257246469,23.475,25.5)) ;
#10972=CARTESIAN_POINT('Origin',(0.25,25.5,25.5)) ;
#10973=CARTESIAN_POINT('',(0.,25.5,30.05)) ;
#10974=CARTESIAN_POINT('Origin',(0.,25.5,25.5)) ;
#10975=CARTESIAN_POINT('',(0.5,25.5,29.55)) ;
#10976=CARTESIAN_POINT('',(0.25,25.5,29.8)) ;
#10977=CARTESIAN_POINT('Origin',(0.5,25.5,25.5)) ;
#10978=CARTESIAN_POINT('Origin',(0.,25.5,25.5)) ;
#10979=CARTESIAN_POINT('',(16.,25.5,29.55)) ;
#10980=CARTESIAN_POINT('',(0.,25.5,29.55)) ;
#10981=CARTESIAN_POINT('',(16.,21.45,25.5)) ;
#10982=CARTESIAN_POINT('Origin',(16.,25.5,25.5)) ;
#10983=CARTESIAN_POINT('Origin',(16.,25.5,25.5)) ;
#10984=CARTESIAN_POINT('Origin',(0.,31.,25.5)) ;
#10985=CARTESIAN_POINT('',(1.6306400674182E-15,20.,25.5)) ;
#10986=CARTESIAN_POINT('Origin',(0.,25.5,25.5)) ;
#10987=CARTESIAN_POINT('Origin',(16.,25.5,25.5)) ;
#10988=CARTESIAN_POINT('',(18.4334855070616,25.5,25.5)) ;
#10989=CARTESIAN_POINT('',(16.,21.45,25.5)) ;
#10990=CARTESIAN_POINT('Origin',(118.,19.5,25.5)) ;
#10991=CARTESIAN_POINT('',(118.,20.5,28.8166247903554)) ;
#10992=CARTESIAN_POINT('',(118.,19.5,25.5)) ;
#10993=CARTESIAN_POINT('Origin',(118.,25.5,25.5)) ;
#10994=CARTESIAN_POINT('',(118.,20.5,22.1833752096446)) ;
#10995=CARTESIAN_POINT('',(118.,20.5,32.5)) ;
#10996=CARTESIAN_POINT('Origin',(118.,25.5,25.5)) ;
#10997=CARTESIAN_POINT('Origin',(106.,20.5,18.5)) ;
#10998=CARTESIAN_POINT('',(106.,20.5,28.8166247903554)) ;
#10999=CARTESIAN_POINT('',(105.75,20.5,28.8166247903554)) ;
#11000=CARTESIAN_POINT('',(106.,20.5,22.1833752096446)) ;
#11001=CARTESIAN_POINT('',(106.,20.5,32.5)) ;
#11002=CARTESIAN_POINT('',(105.75,20.5,22.1833752096446)) ;
#11003=CARTESIAN_POINT('Origin',(106.,19.5,25.5)) ;
#11004=CARTESIAN_POINT('',(106.,19.5,25.5)) ;
#11005=CARTESIAN_POINT('Origin',(106.,25.5,25.5)) ;
#11006=CARTESIAN_POINT('Origin',(106.,25.5,25.5)) ;
#11007=CARTESIAN_POINT('Origin',(106.,31.5,25.5)) ;
#11008=CARTESIAN_POINT('',(106.,30.5,28.8166247903554)) ;
#11009=CARTESIAN_POINT('',(106.,30.5,22.1833752096446)) ;
#11010=CARTESIAN_POINT('Origin',(106.,25.5,25.5)) ;
#11011=CARTESIAN_POINT('',(106.,30.5,32.5)) ;
#11012=CARTESIAN_POINT('Origin',(106.,30.5,32.5)) ;
#11013=CARTESIAN_POINT('',(118.,30.5,28.8166247903554)) ;
#11014=CARTESIAN_POINT('',(105.75,30.5,28.8166247903554)) ;
#11015=CARTESIAN_POINT('',(118.,30.5,22.1833752096446)) ;
#11016=CARTESIAN_POINT('',(118.,30.5,32.5)) ;
#11017=CARTESIAN_POINT('',(105.75,30.5,22.1833752096446)) ;
#11018=CARTESIAN_POINT('Origin',(118.,31.5,25.5)) ;
#11019=CARTESIAN_POINT('Origin',(118.,25.5,25.5)) ;
#11020=CARTESIAN_POINT('Origin',(12.,19.8431457505076,19.8431457505076)) ;
#11021=CARTESIAN_POINT('',(92.,21.2911524926819,19.0520854022295)) ;
#11022=CARTESIAN_POINT('',(91.7,21.1239700652888,18.802958712199)) ;
#11023=CARTESIAN_POINT('Ctrl Pts',(92.,21.2911524926819,19.0520854022295)) ;
#11024=CARTESIAN_POINT('Ctrl Pts',(91.9567026846615,21.2703306474521,19.0139717837895)) ;
#11025=CARTESIAN_POINT('Ctrl Pts',(91.9139415332125,21.2483235990085,18.9772740185191)) ;
#11026=CARTESIAN_POINT('Ctrl Pts',(91.8156742489856,21.1946634967733,18.8949511627776)) ;
#11027=CARTESIAN_POINT('Ctrl Pts',(91.7581599879312,21.1608316055721,18.8483478156355)) ;
#11028=CARTESIAN_POINT('Ctrl Pts',(91.7,21.1239700652888,18.802958712199)) ;
#11029=CARTESIAN_POINT('',(92.,19.0520854022295,21.2911524926819)) ;
#11030=CARTESIAN_POINT('Origin',(92.,19.8431457505076,19.8431457505076)) ;
#11031=CARTESIAN_POINT('',(91.7,18.802958712199,21.1239700652888)) ;
#11032=CARTESIAN_POINT('Ctrl Pts',(91.7,18.802958712199,21.1239700652888)) ;
#11033=CARTESIAN_POINT('Ctrl Pts',(91.7581599873228,18.8483478151607,21.1608316051865)) ;
#11034=CARTESIAN_POINT('Ctrl Pts',(91.8156742480668,18.8949511620079,21.1946634962716)) ;
#11035=CARTESIAN_POINT('Ctrl Pts',(91.872005365357,18.9421422335728,21.2254238203876)) ;
#11036=CARTESIAN_POINT('Ctrl Pts',(91.9139415332125,18.9772740185191,21.2483235990085)) ;
#11037=CARTESIAN_POINT('Ctrl Pts',(91.9567026846615,19.0139717837895,21.2703306474521)) ;
#11038=CARTESIAN_POINT('Ctrl Pts',(92.,19.0520854022295,21.2911524926819)) ;
#11039=CARTESIAN_POINT('',(12.3,18.802958712199,21.1239700652888)) ;
#11040=CARTESIAN_POINT('',(12.,18.802958712199,21.1239700652888)) ;
#11041=CARTESIAN_POINT('',(12.,19.0520854022295,21.2911524926819)) ;
#11042=CARTESIAN_POINT('Ctrl Pts',(12.,19.0520854022295,21.2911524926819)) ;
#11043=CARTESIAN_POINT('Ctrl Pts',(12.0432973155239,19.0139717836263,21.2703306473629)) ;
#11044=CARTESIAN_POINT('Ctrl Pts',(12.0860584670469,18.9772740183018,21.2483235988669)) ;
#11045=CARTESIAN_POINT('Ctrl Pts',(12.127994634643,18.9421422335728,21.2254238203876)) ;
#11046=CARTESIAN_POINT('Ctrl Pts',(12.1843257510144,18.8949511627776,21.1946634967733)) ;
#11047=CARTESIAN_POINT('Ctrl Pts',(12.2418400120688,18.8483478156355,21.1608316055721)) ;
#11048=CARTESIAN_POINT('Ctrl Pts',(12.3,18.802958712199,21.1239700652888)) ;
#11049=CARTESIAN_POINT('',(12.,21.2911524926819,19.0520854022295)) ;
#11050=CARTESIAN_POINT('Origin',(12.,19.8431457505076,19.8431457505076)) ;
#11051=CARTESIAN_POINT('',(12.3,21.1239700652888,18.802958712199)) ;
#11052=CARTESIAN_POINT('Ctrl Pts',(12.3,21.1239700652888,18.802958712199)) ;
#11053=CARTESIAN_POINT('Ctrl Pts',(12.2418400120688,21.1608316055721,18.8483478156355)) ;
#11054=CARTESIAN_POINT('Ctrl Pts',(12.1843257510144,21.1946634967733,18.8949511627776)) ;
#11055=CARTESIAN_POINT('Ctrl Pts',(12.0860584667875,21.2483235990085,18.9772740185191)) ;
#11056=CARTESIAN_POINT('Ctrl Pts',(12.0432973153384,21.2703306474521,19.0139717837895)) ;
#11057=CARTESIAN_POINT('Ctrl Pts',(12.,21.2911524926819,19.0520854022295)) ;
#11058=CARTESIAN_POINT('',(12.,21.1239700652888,18.802958712199)) ;
#11059=CARTESIAN_POINT('Origin',(12.,31.1568542494924,19.8431457505076)) ;
#11060=CARTESIAN_POINT('',(92.,31.9479145977705,21.2911524926819)) ;
#11061=CARTESIAN_POINT('',(91.7,32.197041287801,21.1239700652888)) ;
#11062=CARTESIAN_POINT('Ctrl Pts',(92.,31.9479145977705,21.2911524926819)) ;
#11063=CARTESIAN_POINT('Ctrl Pts',(91.9567026846615,31.9860282162105,21.2703306474521)) ;
#11064=CARTESIAN_POINT('Ctrl Pts',(91.9139415332125,32.0227259814809,21.2483235990085)) ;
#11065=CARTESIAN_POINT('Ctrl Pts',(91.8156742489856,32.1050488372224,21.1946634967733)) ;
#11066=CARTESIAN_POINT('Ctrl Pts',(91.7581599879312,32.1516521843645,21.1608316055721)) ;
#11067=CARTESIAN_POINT('Ctrl Pts',(91.7,32.197041287801,21.1239700652888)) ;
#11068=CARTESIAN_POINT('',(92.,29.7088475073181,19.0520854022295)) ;
#11069=CARTESIAN_POINT('Origin',(92.,31.1568542494924,19.8431457505076)) ;
#11070=CARTESIAN_POINT('',(91.7,29.8760299347112,18.802958712199)) ;
#11071=CARTESIAN_POINT('Ctrl Pts',(91.7,29.8760299347112,18.802958712199)) ;
#11072=CARTESIAN_POINT('Ctrl Pts',(91.7581599873228,29.8391683948135,18.8483478151607)) ;
#11073=CARTESIAN_POINT('Ctrl Pts',(91.8156742480668,29.8053365037284,18.8949511620079)) ;
#11074=CARTESIAN_POINT('Ctrl Pts',(91.872005365357,29.7745761796124,18.9421422335728)) ;
#11075=CARTESIAN_POINT('Ctrl Pts',(91.9139415332125,29.7516764009915,18.9772740185191)) ;
#11076=CARTESIAN_POINT('Ctrl Pts',(91.9567026846615,29.7296693525479,19.0139717837895)) ;
#11077=CARTESIAN_POINT('Ctrl Pts',(92.,29.7088475073181,19.0520854022295)) ;
#11078=CARTESIAN_POINT('',(12.3,29.8760299347112,18.802958712199)) ;
#11079=CARTESIAN_POINT('',(12.,29.8760299347112,18.802958712199)) ;
#11080=CARTESIAN_POINT('',(12.,29.7088475073181,19.0520854022295)) ;
#11081=CARTESIAN_POINT('Ctrl Pts',(12.,29.7088475073181,19.0520854022295)) ;
#11082=CARTESIAN_POINT('Ctrl Pts',(12.0432973155239,29.7296693526371,19.0139717836263)) ;
#11083=CARTESIAN_POINT('Ctrl Pts',(12.0860584670469,29.7516764011331,18.9772740183018)) ;
#11084=CARTESIAN_POINT('Ctrl Pts',(12.127994634643,29.7745761796124,18.9421422335728)) ;
#11085=CARTESIAN_POINT('Ctrl Pts',(12.1843257510144,29.8053365032267,18.8949511627776)) ;
#11086=CARTESIAN_POINT('Ctrl Pts',(12.2418400120688,29.8391683944279,18.8483478156355)) ;
#11087=CARTESIAN_POINT('Ctrl Pts',(12.3,29.8760299347112,18.802958712199)) ;
#11088=CARTESIAN_POINT('',(12.,31.9479145977705,21.2911524926819)) ;
#11089=CARTESIAN_POINT('Origin',(12.,31.1568542494924,19.8431457505076)) ;
#11090=CARTESIAN_POINT('',(12.3,32.197041287801,21.1239700652888)) ;
#11091=CARTESIAN_POINT('Ctrl Pts',(12.3,32.197041287801,21.1239700652888)) ;
#11092=CARTESIAN_POINT('Ctrl Pts',(12.2418400120688,32.1516521843645,21.1608316055721)) ;
#11093=CARTESIAN_POINT('Ctrl Pts',(12.1843257510144,32.1050488372224,21.1946634967733)) ;
#11094=CARTESIAN_POINT('Ctrl Pts',(12.0860584667875,32.0227259814809,21.2483235990085)) ;
#11095=CARTESIAN_POINT('Ctrl Pts',(12.0432973153384,31.9860282162105,21.2703306474521)) ;
#11096=CARTESIAN_POINT('Ctrl Pts',(12.,31.9479145977705,21.2911524926819)) ;
#11097=CARTESIAN_POINT('',(12.,32.197041287801,21.1239700652888)) ;
#11098=CARTESIAN_POINT('Origin',(12.,31.1568542494924,31.1568542494924)) ;
#11099=CARTESIAN_POINT('',(91.7,32.197041287801,29.8760299347112)) ;
#11100=CARTESIAN_POINT('',(92.,31.9479145977705,29.7088475073181)) ;
#11101=CARTESIAN_POINT('Ctrl Pts',(91.7,32.197041287801,29.8760299347112)) ;
#11102=CARTESIAN_POINT('Ctrl Pts',(91.7581599873228,32.1516521848393,29.8391683948135)) ;
#11103=CARTESIAN_POINT('Ctrl Pts',(91.8156742480668,32.1050488379921,29.8053365037284)) ;
#11104=CARTESIAN_POINT('Ctrl Pts',(91.872005365357,32.0578577664272,29.7745761796124)) ;
#11105=CARTESIAN_POINT('Ctrl Pts',(91.9139415332125,32.0227259814809,29.7516764009914)) ;
#11106=CARTESIAN_POINT('Ctrl Pts',(91.9567026846615,31.9860282162105,29.7296693525479)) ;
#11107=CARTESIAN_POINT('Ctrl Pts',(92.,31.9479145977705,29.7088475073181)) ;
#11108=CARTESIAN_POINT('',(12.3,32.197041287801,29.8760299347112)) ;
#11109=CARTESIAN_POINT('',(12.,32.197041287801,29.8760299347112)) ;
#11110=CARTESIAN_POINT('',(12.,31.9479145977705,29.7088475073181)) ;
#11111=CARTESIAN_POINT('Ctrl Pts',(12.,31.9479145977705,29.7088475073181)) ;
#11112=CARTESIAN_POINT('Ctrl Pts',(12.0432973155239,31.9860282163737,29.7296693526371)) ;
#11113=CARTESIAN_POINT('Ctrl Pts',(12.0860584670469,32.0227259816982,29.7516764011331)) ;
#11114=CARTESIAN_POINT('Ctrl Pts',(12.127994634643,32.0578577664272,29.7745761796124)) ;
#11115=CARTESIAN_POINT('Ctrl Pts',(12.1843257510144,32.1050488372224,29.8053365032267)) ;
#11116=CARTESIAN_POINT('Ctrl Pts',(12.2418400120688,32.1516521843645,29.8391683944279)) ;
#11117=CARTESIAN_POINT('Ctrl Pts',(12.3,32.197041287801,29.8760299347112)) ;
#11118=CARTESIAN_POINT('',(12.,29.7088475073181,31.9479145977705)) ;
#11119=CARTESIAN_POINT('Origin',(12.,31.1568542494924,31.1568542494924)) ;
#11120=CARTESIAN_POINT('',(12.3,29.8760299347112,32.197041287801)) ;
#11121=CARTESIAN_POINT('Ctrl Pts',(12.3,29.8760299347112,32.197041287801)) ;
#11122=CARTESIAN_POINT('Ctrl Pts',(12.2418400120688,29.8391683944279,32.1516521843645)) ;
#11123=CARTESIAN_POINT('Ctrl Pts',(12.1843257510144,29.8053365032267,32.1050488372224)) ;
#11124=CARTESIAN_POINT('Ctrl Pts',(12.0860584667875,29.7516764009915,32.0227259814809)) ;
#11125=CARTESIAN_POINT('Ctrl Pts',(12.0432973153384,29.7296693525479,31.9860282162105)) ;
#11126=CARTESIAN_POINT('Ctrl Pts',(12.,29.7088475073181,31.9479145977705)) ;
#11127=CARTESIAN_POINT('',(91.7,29.8760299347112,32.197041287801)) ;
#11128=CARTESIAN_POINT('',(12.,29.8760299347112,32.197041287801)) ;
#11129=CARTESIAN_POINT('',(92.,29.7088475073181,31.9479145977705)) ;
#11130=CARTESIAN_POINT('Ctrl Pts',(92.,29.7088475073181,31.9479145977705)) ;
#11131=CARTESIAN_POINT('Ctrl Pts',(91.9567026846615,29.7296693525479,31.9860282162105)) ;
#11132=CARTESIAN_POINT('Ctrl Pts',(91.9139415332125,29.7516764009915,32.0227259814809)) ;
#11133=CARTESIAN_POINT('Ctrl Pts',(91.8156742489856,29.8053365032267,32.1050488372224)) ;
#11134=CARTESIAN_POINT('Ctrl Pts',(91.7581599879312,29.8391683944279,32.1516521843645)) ;
#11135=CARTESIAN_POINT('Ctrl Pts',(91.7,29.8760299347112,32.197041287801)) ;
#11136=CARTESIAN_POINT('Origin',(92.,31.1568542494924,31.1568542494924)) ;
#11137=CARTESIAN_POINT('Origin',(12.,19.8431457505076,31.1568542494924)) ;
#11138=CARTESIAN_POINT('',(91.7,21.1239700652888,32.197041287801)) ;
#11139=CARTESIAN_POINT('',(92.,21.2911524926819,31.9479145977705)) ;
#11140=CARTESIAN_POINT('Ctrl Pts',(91.7,21.1239700652888,32.197041287801)) ;
#11141=CARTESIAN_POINT('Ctrl Pts',(91.7581599873228,21.1608316051865,32.1516521848393)) ;
#11142=CARTESIAN_POINT('Ctrl Pts',(91.8156742480668,21.1946634962716,32.1050488379921)) ;
#11143=CARTESIAN_POINT('Ctrl Pts',(91.872005365357,21.2254238203876,32.0578577664272)) ;
#11144=CARTESIAN_POINT('Ctrl Pts',(91.9139415332125,21.2483235990085,32.0227259814809)) ;
#11145=CARTESIAN_POINT('Ctrl Pts',(91.9567026846616,21.2703306474521,31.9860282162104)) ;
#11146=CARTESIAN_POINT('Ctrl Pts',(92.,21.2911524926819,31.9479145977705)) ;
#11147=CARTESIAN_POINT('',(12.3,21.1239700652888,32.197041287801)) ;
#11148=CARTESIAN_POINT('',(12.,21.1239700652888,32.197041287801)) ;
#11149=CARTESIAN_POINT('',(12.,21.2911524926819,31.9479145977705)) ;
#11150=CARTESIAN_POINT('Ctrl Pts',(12.,21.2911524926819,31.9479145977705)) ;
#11151=CARTESIAN_POINT('Ctrl Pts',(12.0432973155239,21.2703306473629,31.9860282163737)) ;
#11152=CARTESIAN_POINT('Ctrl Pts',(12.0860584670469,21.2483235988669,32.0227259816982)) ;
#11153=CARTESIAN_POINT('Ctrl Pts',(12.127994634643,21.2254238203876,32.0578577664272)) ;
#11154=CARTESIAN_POINT('Ctrl Pts',(12.1843257510144,21.1946634967733,32.1050488372224)) ;
#11155=CARTESIAN_POINT('Ctrl Pts',(12.2418400120688,21.1608316055721,32.1516521843645)) ;
#11156=CARTESIAN_POINT('Ctrl Pts',(12.3,21.1239700652888,32.197041287801)) ;
#11157=CARTESIAN_POINT('',(12.,19.0520854022295,29.7088475073181)) ;
#11158=CARTESIAN_POINT('Origin',(12.,19.8431457505076,31.1568542494924)) ;
#11159=CARTESIAN_POINT('',(12.3,18.802958712199,29.8760299347112)) ;
#11160=CARTESIAN_POINT('Ctrl Pts',(12.3,18.802958712199,29.8760299347112)) ;
#11161=CARTESIAN_POINT('Ctrl Pts',(12.2418400120688,18.8483478156355,29.8391683944279)) ;
#11162=CARTESIAN_POINT('Ctrl Pts',(12.1843257510144,18.8949511627776,29.8053365032267)) ;
#11163=CARTESIAN_POINT('Ctrl Pts',(12.0860584667875,18.9772740185191,29.7516764009915)) ;
#11164=CARTESIAN_POINT('Ctrl Pts',(12.0432973153384,19.0139717837895,29.7296693525479)) ;
#11165=CARTESIAN_POINT('Ctrl Pts',(12.,19.0520854022295,29.7088475073181)) ;
#11166=CARTESIAN_POINT('',(91.7,18.802958712199,29.8760299347112)) ;
#11167=CARTESIAN_POINT('',(12.,18.802958712199,29.8760299347112)) ;
#11168=CARTESIAN_POINT('',(92.,19.0520854022295,29.7088475073181)) ;
#11169=CARTESIAN_POINT('Ctrl Pts',(92.,19.0520854022295,29.7088475073181)) ;
#11170=CARTESIAN_POINT('Ctrl Pts',(91.9567026846615,19.0139717837895,29.7296693525479)) ;
#11171=CARTESIAN_POINT('Ctrl Pts',(91.9139415332125,18.9772740185191,29.7516764009915)) ;
#11172=CARTESIAN_POINT('Ctrl Pts',(91.8156742489856,18.8949511627776,29.8053365032267)) ;
#11173=CARTESIAN_POINT('Ctrl Pts',(91.7581599879312,18.8483478156355,29.8391683944279)) ;
#11174=CARTESIAN_POINT('Ctrl Pts',(91.7,18.802958712199,29.8760299347112)) ;
#11175=CARTESIAN_POINT('Origin',(92.,19.8431457505076,31.1568542494924)) ;
#11176=CARTESIAN_POINT('Origin',(91.85,25.5,25.5)) ;
#11177=CARTESIAN_POINT('Origin',(91.7,25.5,25.5)) ;
#11178=CARTESIAN_POINT('Origin',(92.,25.5,25.5)) ;
#11179=CARTESIAN_POINT('Origin',(91.85,25.5,25.5)) ;
#11180=CARTESIAN_POINT('Origin',(91.7,25.5,25.5)) ;
#11181=CARTESIAN_POINT('Origin',(92.,25.5,25.5)) ;
#11182=CARTESIAN_POINT('Origin',(91.85,25.5,25.5)) ;
#11183=CARTESIAN_POINT('Origin',(92.,25.5,25.5)) ;
#11184=CARTESIAN_POINT('Origin',(91.7,25.5,25.5)) ;
#11185=CARTESIAN_POINT('Origin',(91.85,25.5,25.5)) ;
#11186=CARTESIAN_POINT('Origin',(91.7,25.5,25.5)) ;
#11187=CARTESIAN_POINT('Origin',(92.,25.5,25.5)) ;
#11188=CARTESIAN_POINT('Origin',(52.,25.5,25.5)) ;
#11189=CARTESIAN_POINT('Origin',(12.3,25.5,25.5)) ;
#11190=CARTESIAN_POINT('Origin',(52.,25.5,25.5)) ;
#11191=CARTESIAN_POINT('Origin',(12.3,25.5,25.5)) ;
#11192=CARTESIAN_POINT('Origin',(52.,25.5,25.5)) ;
#11193=CARTESIAN_POINT('Origin',(12.3,25.5,25.5)) ;
#11194=CARTESIAN_POINT('Origin',(52.,25.5,25.5)) ;
#11195=CARTESIAN_POINT('Origin',(12.3,25.5,25.5)) ;
#11196=CARTESIAN_POINT('Origin',(12.15,25.5,25.5)) ;
#11197=CARTESIAN_POINT('Origin',(12.,25.5,25.5)) ;
#11198=CARTESIAN_POINT('Origin',(12.15,25.5,25.5)) ;
#11199=CARTESIAN_POINT('Origin',(12.,25.5,25.5)) ;
#11200=CARTESIAN_POINT('Origin',(12.15,25.5,25.5)) ;
#11201=CARTESIAN_POINT('Origin',(12.,25.5,25.5)) ;
#11202=CARTESIAN_POINT('Origin',(12.15,25.5,25.5)) ;
#11203=CARTESIAN_POINT('Origin',(12.,25.5,25.5)) ;
#11204=CARTESIAN_POINT('Origin',(12.,33.2,25.5)) ;
#11205=CARTESIAN_POINT('',(12.,19.5,25.5)) ;
#11206=CARTESIAN_POINT('Origin',(12.,25.5,25.5)) ;
#11207=CARTESIAN_POINT('Origin',(0.250000000000004,25.5,25.5)) ;
#11208=CARTESIAN_POINT('',(0.500000000000006,19.5,25.5)) ;
#11209=CARTESIAN_POINT('Origin',(0.500000000000007,25.5,25.5)) ;
#11210=CARTESIAN_POINT('',(0.250000000000004,19.75,25.5)) ;
#11211=CARTESIAN_POINT('Origin',(6.25,25.5,25.5)) ;
#11212=CARTESIAN_POINT('',(6.25,19.5,25.5)) ;
#11213=CARTESIAN_POINT('Origin',(92.,31.5,25.5)) ;
#11214=CARTESIAN_POINT('',(92.,19.5,25.5)) ;
#11215=CARTESIAN_POINT('Origin',(92.,25.5,25.5)) ;
#11216=CARTESIAN_POINT('Origin',(105.75,25.5,25.5)) ;
#11217=CARTESIAN_POINT('',(119.5,19.5,25.5)) ;
#11218=CARTESIAN_POINT('Origin',(119.5,25.5,25.5)) ;
#11219=CARTESIAN_POINT('',(105.75,19.5,25.5)) ;
#11220=CARTESIAN_POINT('',(105.75,19.5,25.5)) ;
#11221=CARTESIAN_POINT('Origin',(119.75,25.5,25.5)) ;
#11222=CARTESIAN_POINT('',(119.75,19.75,25.5)) ;
#16926=UNCERTAINTY_MEASURE_WITH_UNIT(LENGTH_MEASURE(0.01),#16943,
'DISTANCE_ACCURACY_VALUE',
'Maximum model space distance between geometric entities at asserted c
onnectivities') ;
#16933=UNCERTAINTY_MEASURE_WITH_UNIT(LENGTH_MEASURE(0.01),#16943,
'DISTANCE_ACCURACY_VALUE',
'Maximum model space distance between geometric entities at asserted c
onnectivities') ;
#16935=(
GEOMETRIC_REPRESENTATION_CONTEXT(3)
GLOBAL_UNCERTAINTY_ASSIGNED_CONTEXT((#16926))
GLOBAL_UNIT_ASSIGNED_CONTEXT((#16943,#16945,#16946))
REPRESENTATION_CONTEXT('','3D')
) ;
#16942=(
GEOMETRIC_REPRESENTATION_CONTEXT(3)
GLOBAL_UNCERTAINTY_ASSIGNED_CONTEXT((#16933))
GLOBAL_UNIT_ASSIGNED_CONTEXT((#16943,#16945,#16946))
REPRESENTATION_CONTEXT('','3D')
) ;
#16943=(
LENGTH_UNIT()
NAMED_UNIT(*)
SI_UNIT(.MILLI.,.METRE.)
) ;
#16945=(
NAMED_UNIT(*)
PLANE_ANGLE_UNIT()
SI_UNIT($,.RADIAN.)
) ;
#16946=(
NAMED_UNIT(*)
SI_UNIT($,.STERADIAN.)
SOLID_ANGLE_UNIT()
) ;
#16948=SHAPE_DEFINITION_REPRESENTATION(#16956,#17019) ;
#16956=PRODUCT_DEFINITION_SHAPE('',$,#17028) ;
#17019=SHAPE_REPRESENTATION('',(#8264),#16935) ;
#17026=PRODUCT_DEFINITION_CONTEXT('part definition',#17052,'design') ;
#17028=PRODUCT_DEFINITION('Ball Spline Shaft No.16 x 120 Stepped D12 Tapped M8',
'Ball Spline Shaft No.16 x 120 Stepped D12 Tapped M8',#17036,#17026) ;
#17036=PRODUCT_DEFINITION_FORMATION('',$,#17055) ;
#17052=APPLICATION_CONTEXT(
'Core Data for Automotive Mechanical Design Process') ;
#17053=PRODUCT_CONTEXT('part definition',#17052,'mechanical') ;
#17055=PRODUCT('Ball Spline Shaft No.16 x 120 Stepped D12 Tapped M8',
'Ball Spline Shaft No.16 x 120 Stepped D12 Tapped M8',$,(#17053)) ;
#17063=PRESENTATION_STYLE_ASSIGNMENT((#17071)) ;
#17071=SURFACE_STYLE_USAGE(.BOTH.,#17079) ;
#17079=SURFACE_SIDE_STYLE('',(#17087)) ;
#17087=SURFACE_STYLE_FILL_AREA(#17095) ;
#17095=FILL_AREA_STYLE(
'MAS-257 Metallic Sheet - Ball Spline Shaft No.16 x 120 Stepped D1',(#17103)) ;
#17103=FILL_AREA_STYLE_COLOUR(
'MAS-257 Metallic Sheet - Ball Spline Shaft No.16 x 120 Stepped D1',#17111) ;
#17111=COLOUR_RGB(
'MAS-257 Metallic Sheet - Ball Spline Shaft No.16 x 120 Stepped D1', 0.66274510, 0.83137255, 0.94901961) ;
ENDSEC;
END-ISO-10303-21;
